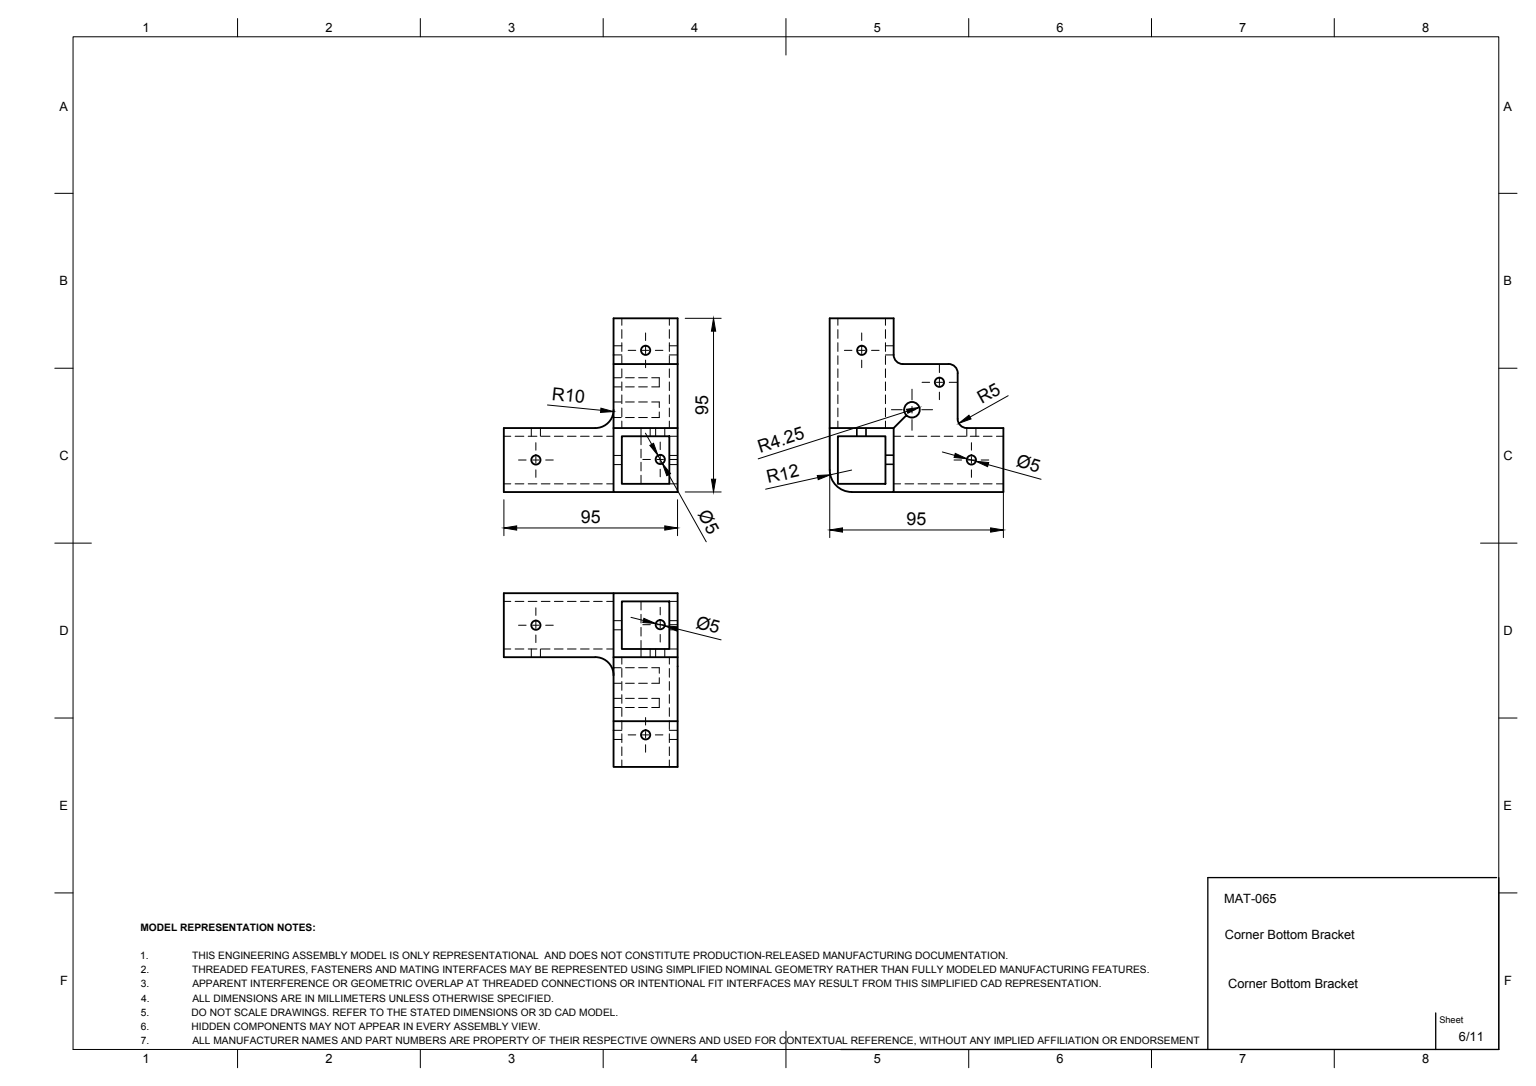
ISO-10303-21;
HEADER;
/* Generated by software containing ST-Developer
 * from STEP Tools, Inc. (www.steptools.com) 
 */

FILE_DESCRIPTION(
/* description */ (
'CAx-IF Rec.Pracs.---Representation and Presentation of Product Manufa
cturing Information (PMI)---4.0---2014-10-13'),
/* implementation_level */ '2;1');

FILE_NAME(
/* name */ 'Corner Bottom Bracket.step',
/* time_stamp */ '2026-11-15T23:28:27-08:00',
/* author */ (''),
/* organization */ (''),
/* preprocessor_version */ 'ST-DEVELOPER v20.2',
/* originating_system */ 'Autodesk Translation Framework v15.17.0.0',
/* authorisation */ '');

FILE_SCHEMA (('AUTOMOTIVE_DESIGN { 1 0 10303 214 3 1 1 }'));
ENDSEC;

DATA;
#10=MECHANICAL_DESIGN_GEOMETRIC_PRESENTATION_REPRESENTATION('',(#197),#7756);
#166=ELLIPSE('',#5063,0.0141421356237309,0.01);
#169=B_SPLINE_CURVE_WITH_KNOTS('',3,(#7622,#7623,#7624,#7625,#7626,#7627),
 .UNSPECIFIED.,.F.,.F.,(4,2,4),(-0.973960746358264,-0.811705326326323,-0.649449906294381),
 .UNSPECIFIED.);
#170=B_SPLINE_CURVE_WITH_KNOTS('',3,(#7661,#7662,#7663,#7664,#7665,#7666),
 .UNSPECIFIED.,.F.,.F.,(4,2,4),(0.649449906294381,0.811705326326323,0.973960746358265),
 .UNSPECIFIED.);
#179=SHAPE_REPRESENTATION_RELATIONSHIP('SRR','None',#7827,#188);
#188=ADVANCED_BREP_SHAPE_REPRESENTATION('',(#206),#7755);
#197=STYLED_ITEM('',(#7878),#206);
#206=MANIFOLD_SOLID_BREP('Body1',#4634);
#246=CYLINDRICAL_SURFACE('',#5062,0.01);
#247=CYLINDRICAL_SURFACE('',#5064,0.012);
#248=CYLINDRICAL_SURFACE('',#5065,0.0025);
#249=CYLINDRICAL_SURFACE('',#5066,0.0025);
#250=CYLINDRICAL_SURFACE('',#5067,0.0025);
#251=CYLINDRICAL_SURFACE('',#5068,0.0025);
#252=CYLINDRICAL_SURFACE('',#5069,0.0025);
#253=CYLINDRICAL_SURFACE('',#5070,0.0025);
#254=CYLINDRICAL_SURFACE('',#5071,0.0025);
#255=CYLINDRICAL_SURFACE('',#5072,0.0025);
#256=CYLINDRICAL_SURFACE('',#5075,0.0025);
#257=CYLINDRICAL_SURFACE('',#5078,0.00425);
#258=CYLINDRICAL_SURFACE('',#5081,0.01);
#259=CYLINDRICAL_SURFACE('',#5082,0.005);
#260=CYLINDRICAL_SURFACE('',#5083,0.005);
#261=CYLINDRICAL_SURFACE('',#5084,0.005);
#262=CYLINDRICAL_SURFACE('',#5092,0.0025);
#263=CYLINDRICAL_SURFACE('',#5093,0.0025);
#342=CIRCLE('',#5005,0.005);
#343=CIRCLE('',#5006,0.005);
#344=CIRCLE('',#5007,0.012);
#345=CIRCLE('',#5008,0.005);
#346=CIRCLE('',#5009,0.0025);
#347=CIRCLE('',#5010,0.0025);
#348=CIRCLE('',#5012,0.0025);
#349=CIRCLE('',#5013,0.0025);
#350=CIRCLE('',#5015,0.0025);
#351=CIRCLE('',#5016,0.0025);
#352=CIRCLE('',#5018,0.012);
#353=CIRCLE('',#5022,0.01);
#354=CIRCLE('',#5024,0.01);
#355=CIRCLE('',#5026,0.005);
#356=CIRCLE('',#5027,0.005);
#357=CIRCLE('',#5028,0.00425);
#358=CIRCLE('',#5029,0.005);
#359=CIRCLE('',#5030,0.0025);
#360=CIRCLE('',#5031,0.0025);
#361=CIRCLE('',#5032,0.0025);
#362=CIRCLE('',#5034,0.0025);
#363=CIRCLE('',#5036,0.0025);
#364=CIRCLE('',#5038,0.0025);
#365=CIRCLE('',#5041,0.0025);
#366=CIRCLE('',#5043,0.0025);
#367=CIRCLE('',#5045,0.0025);
#368=CIRCLE('',#5047,0.0025);
#369=CIRCLE('',#5049,0.0025);
#370=CIRCLE('',#5051,0.0025);
#371=CIRCLE('',#5054,0.0025);
#372=CIRCLE('',#5056,0.0025);
#373=CIRCLE('',#5060,0.0025);
#374=CIRCLE('',#5076,0.0025);
#375=CIRCLE('',#5079,0.00425);
#376=CIRCLE('',#5086,0.0025);
#377=CIRCLE('',#5088,0.0025);
#429=FACE_BOUND('',#917,.T.);
#430=FACE_BOUND('',#918,.T.);
#431=FACE_BOUND('',#919,.T.);
#432=FACE_BOUND('',#923,.T.);
#433=FACE_BOUND('',#925,.T.);
#434=FACE_BOUND('',#927,.T.);
#435=FACE_BOUND('',#931,.T.);
#436=FACE_BOUND('',#932,.T.);
#437=FACE_BOUND('',#933,.T.);
#438=FACE_BOUND('',#935,.T.);
#439=FACE_BOUND('',#937,.T.);
#440=FACE_BOUND('',#939,.T.);
#441=FACE_BOUND('',#942,.T.);
#442=FACE_BOUND('',#944,.T.);
#443=FACE_BOUND('',#946,.T.);
#444=FACE_BOUND('',#948,.T.);
#445=FACE_BOUND('',#950,.T.);
#446=FACE_BOUND('',#952,.T.);
#447=FACE_BOUND('',#955,.T.);
#448=FACE_BOUND('',#957,.T.);
#449=FACE_BOUND('',#961,.T.);
#450=FACE_BOUND('',#984,.T.);
#451=FACE_BOUND('',#986,.T.);
#632=FACE_OUTER_BOUND('',#916,.T.);
#633=FACE_OUTER_BOUND('',#920,.T.);
#634=FACE_OUTER_BOUND('',#921,.T.);
#635=FACE_OUTER_BOUND('',#922,.T.);
#636=FACE_OUTER_BOUND('',#924,.T.);
#637=FACE_OUTER_BOUND('',#926,.T.);
#638=FACE_OUTER_BOUND('',#928,.T.);
#639=FACE_OUTER_BOUND('',#929,.T.);
#640=FACE_OUTER_BOUND('',#930,.T.);
#641=FACE_OUTER_BOUND('',#934,.T.);
#642=FACE_OUTER_BOUND('',#936,.T.);
#643=FACE_OUTER_BOUND('',#938,.T.);
#644=FACE_OUTER_BOUND('',#940,.T.);
#645=FACE_OUTER_BOUND('',#941,.T.);
#646=FACE_OUTER_BOUND('',#943,.T.);
#647=FACE_OUTER_BOUND('',#945,.T.);
#648=FACE_OUTER_BOUND('',#947,.T.);
#649=FACE_OUTER_BOUND('',#949,.T.);
#650=FACE_OUTER_BOUND('',#951,.T.);
#651=FACE_OUTER_BOUND('',#953,.T.);
#652=FACE_OUTER_BOUND('',#954,.T.);
#653=FACE_OUTER_BOUND('',#956,.T.);
#654=FACE_OUTER_BOUND('',#958,.T.);
#655=FACE_OUTER_BOUND('',#959,.T.);
#656=FACE_OUTER_BOUND('',#960,.T.);
#657=FACE_OUTER_BOUND('',#962,.T.);
#658=FACE_OUTER_BOUND('',#963,.T.);
#659=FACE_OUTER_BOUND('',#964,.T.);
#660=FACE_OUTER_BOUND('',#965,.T.);
#661=FACE_OUTER_BOUND('',#966,.T.);
#662=FACE_OUTER_BOUND('',#967,.T.);
#663=FACE_OUTER_BOUND('',#968,.T.);
#664=FACE_OUTER_BOUND('',#969,.T.);
#665=FACE_OUTER_BOUND('',#970,.T.);
#666=FACE_OUTER_BOUND('',#971,.T.);
#667=FACE_OUTER_BOUND('',#972,.T.);
#668=FACE_OUTER_BOUND('',#973,.T.);
#669=FACE_OUTER_BOUND('',#974,.T.);
#670=FACE_OUTER_BOUND('',#975,.T.);
#671=FACE_OUTER_BOUND('',#976,.T.);
#672=FACE_OUTER_BOUND('',#977,.T.);
#673=FACE_OUTER_BOUND('',#978,.T.);
#674=FACE_OUTER_BOUND('',#979,.T.);
#675=FACE_OUTER_BOUND('',#980,.T.);
#676=FACE_OUTER_BOUND('',#981,.T.);
#677=FACE_OUTER_BOUND('',#982,.T.);
#678=FACE_OUTER_BOUND('',#983,.T.);
#679=FACE_OUTER_BOUND('',#985,.T.);
#680=FACE_OUTER_BOUND('',#987,.T.);
#681=FACE_OUTER_BOUND('',#988,.T.);
#682=FACE_OUTER_BOUND('',#989,.T.);
#683=FACE_OUTER_BOUND('',#990,.T.);
#684=FACE_OUTER_BOUND('',#991,.T.);
#916=EDGE_LOOP('',(#3939,#3940,#3941,#3942,#3943,#3944,#3945,#3946,#3947,
#3948,#3949,#3950));
#917=EDGE_LOOP('',(#3951));
#918=EDGE_LOOP('',(#3952));
#919=EDGE_LOOP('',(#3953,#3954,#3955,#3956));
#920=EDGE_LOOP('',(#3957,#3958,#3959,#3960,#3961,#3962,#3963));
#921=EDGE_LOOP('',(#3964,#3965,#3966,#3967,#3968,#3969,#3970));
#922=EDGE_LOOP('',(#3971,#3972,#3973,#3974,#3975));
#923=EDGE_LOOP('',(#3976,#3977,#3978,#3979));
#924=EDGE_LOOP('',(#3980,#3981,#3982,#3983));
#925=EDGE_LOOP('',(#3984,#3985,#3986,#3987));
#926=EDGE_LOOP('',(#3988,#3989,#3990,#3991));
#927=EDGE_LOOP('',(#3992,#3993,#3994,#3995));
#928=EDGE_LOOP('',(#3996,#3997,#3998,#3999,#4000,#4001,#4002));
#929=EDGE_LOOP('',(#4003,#4004,#4005,#4006,#4007,#4008,#4009));
#930=EDGE_LOOP('',(#4010,#4011,#4012,#4013,#4014,#4015,#4016,#4017,#4018,
#4019,#4020,#4021,#4022,#4023));
#931=EDGE_LOOP('',(#4024));
#932=EDGE_LOOP('',(#4025));
#933=EDGE_LOOP('',(#4026));
#934=EDGE_LOOP('',(#4027,#4028,#4029,#4030));
#935=EDGE_LOOP('',(#4031));
#936=EDGE_LOOP('',(#4032,#4033,#4034,#4035));
#937=EDGE_LOOP('',(#4036));
#938=EDGE_LOOP('',(#4037,#4038,#4039,#4040));
#939=EDGE_LOOP('',(#4041));
#940=EDGE_LOOP('',(#4042,#4043,#4044,#4045));
#941=EDGE_LOOP('',(#4046,#4047,#4048,#4049));
#942=EDGE_LOOP('',(#4050));
#943=EDGE_LOOP('',(#4051,#4052,#4053,#4054));
#944=EDGE_LOOP('',(#4055));
#945=EDGE_LOOP('',(#4056,#4057,#4058,#4059));
#946=EDGE_LOOP('',(#4060));
#947=EDGE_LOOP('',(#4061,#4062,#4063,#4064));
#948=EDGE_LOOP('',(#4065));
#949=EDGE_LOOP('',(#4066,#4067,#4068,#4069));
#950=EDGE_LOOP('',(#4070));
#951=EDGE_LOOP('',(#4071,#4072,#4073,#4074));
#952=EDGE_LOOP('',(#4075));
#953=EDGE_LOOP('',(#4076,#4077,#4078,#4079));
#954=EDGE_LOOP('',(#4080,#4081,#4082,#4083));
#955=EDGE_LOOP('',(#4084));
#956=EDGE_LOOP('',(#4085,#4086,#4087,#4088));
#957=EDGE_LOOP('',(#4089));
#958=EDGE_LOOP('',(#4090,#4091,#4092,#4093));
#959=EDGE_LOOP('',(#4094,#4095,#4096,#4097));
#960=EDGE_LOOP('',(#4098,#4099,#4100,#4101));
#961=EDGE_LOOP('',(#4102));
#962=EDGE_LOOP('',(#4103,#4104,#4105,#4106));
#963=EDGE_LOOP('',(#4107,#4108,#4109,#4110,#4111));
#964=EDGE_LOOP('',(#4112,#4113,#4114,#4115));
#965=EDGE_LOOP('',(#4116,#4117,#4118,#4119));
#966=EDGE_LOOP('',(#4120,#4121,#4122,#4123));
#967=EDGE_LOOP('',(#4124,#4125,#4126,#4127));
#968=EDGE_LOOP('',(#4128,#4129,#4130,#4131));
#969=EDGE_LOOP('',(#4132,#4133,#4134,#4135));
#970=EDGE_LOOP('',(#4136,#4137,#4138,#4139,#4140));
#971=EDGE_LOOP('',(#4141,#4142,#4143,#4144));
#972=EDGE_LOOP('',(#4145,#4146,#4147,#4148,#4149));
#973=EDGE_LOOP('',(#4150,#4151,#4152,#4153));
#974=EDGE_LOOP('',(#4154,#4155,#4156,#4157));
#975=EDGE_LOOP('',(#4158,#4159,#4160,#4161));
#976=EDGE_LOOP('',(#4162));
#977=EDGE_LOOP('',(#4163,#4164,#4165,#4166,#4167,#4168));
#978=EDGE_LOOP('',(#4169));
#979=EDGE_LOOP('',(#4170,#4171,#4172,#4173,#4174));
#980=EDGE_LOOP('',(#4175,#4176,#4177,#4178,#4179));
#981=EDGE_LOOP('',(#4180,#4181,#4182,#4183,#4184));
#982=EDGE_LOOP('',(#4185,#4186,#4187,#4188));
#983=EDGE_LOOP('',(#4189,#4190,#4191,#4192));
#984=EDGE_LOOP('',(#4193));
#985=EDGE_LOOP('',(#4194,#4195,#4196,#4197));
#986=EDGE_LOOP('',(#4198));
#987=EDGE_LOOP('',(#4199,#4200,#4201,#4202));
#988=EDGE_LOOP('',(#4203,#4204,#4205,#4206));
#989=EDGE_LOOP('',(#4207,#4208,#4209,#4210));
#990=EDGE_LOOP('',(#4211,#4212,#4213,#4214));
#991=EDGE_LOOP('',(#4215,#4216,#4217,#4218));
#1384=LINE('',#7405,#1877);
#1385=LINE('',#7409,#1878);
#1386=LINE('',#7413,#1879);
#1387=LINE('',#7415,#1880);
#1388=LINE('',#7417,#1881);
#1389=LINE('',#7421,#1882);
#1390=LINE('',#7423,#1883);
#1391=LINE('',#7425,#1884);
#1392=LINE('',#7433,#1885);
#1393=LINE('',#7435,#1886);
#1394=LINE('',#7437,#1887);
#1395=LINE('',#7438,#1888);
#1396=LINE('',#7442,#1889);
#1397=LINE('',#7444,#1890);
#1398=LINE('',#7448,#1891);
#1399=LINE('',#7449,#1892);
#1400=LINE('',#7452,#1893);
#1401=LINE('',#7457,#1894);
#1402=LINE('',#7459,#1895);
#1403=LINE('',#7460,#1896);
#1404=LINE('',#7464,#1897);
#1405=LINE('',#7468,#1898);
#1406=LINE('',#7470,#1899);
#1407=LINE('',#7471,#1900);
#1408=LINE('',#7474,#1901);
#1409=LINE('',#7476,#1902);
#1410=LINE('',#7478,#1903);
#1411=LINE('',#7479,#1904);
#1412=LINE('',#7482,#1905);
#1413=LINE('',#7483,#1906);
#1414=LINE('',#7486,#1907);
#1415=LINE('',#7488,#1908);
#1416=LINE('',#7490,#1909);
#1417=LINE('',#7491,#1910);
#1418=LINE('',#7494,#1911);
#1419=LINE('',#7495,#1912);
#1420=LINE('',#7498,#1913);
#1421=LINE('',#7500,#1914);
#1422=LINE('',#7502,#1915);
#1423=LINE('',#7503,#1916);
#1424=LINE('',#7505,#1917);
#1425=LINE('',#7507,#1918);
#1426=LINE('',#7510,#1919);
#1427=LINE('',#7512,#1920);
#1428=LINE('',#7514,#1921);
#1429=LINE('',#7517,#1922);
#1430=LINE('',#7521,#1923);
#1431=LINE('',#7525,#1924);
#1432=LINE('',#7528,#1925);
#1433=LINE('',#7531,#1926);
#1434=LINE('',#7541,#1927);
#1435=LINE('',#7542,#1928);
#1436=LINE('',#7546,#1929);
#1437=LINE('',#7551,#1930);
#1438=LINE('',#7553,#1931);
#1439=LINE('',#7554,#1932);
#1440=LINE('',#7559,#1933);
#1441=LINE('',#7560,#1934);
#1442=LINE('',#7563,#1935);
#1443=LINE('',#7564,#1936);
#1444=LINE('',#7568,#1937);
#1445=LINE('',#7576,#1938);
#1446=LINE('',#7578,#1939);
#1447=LINE('',#7579,#1940);
#1448=LINE('',#7584,#1941);
#1449=LINE('',#7585,#1942);
#1450=LINE('',#7590,#1943);
#1451=LINE('',#7591,#1944);
#1452=LINE('',#7595,#1945);
#1453=LINE('',#7601,#1946);
#1454=LINE('',#7603,#1947);
#1455=LINE('',#7604,#1948);
#1456=LINE('',#7609,#1949);
#1457=LINE('',#7610,#1950);
#1458=LINE('',#7613,#1951);
#1459=LINE('',#7614,#1952);
#1460=LINE('',#7616,#1953);
#1461=LINE('',#7631,#1954);
#1462=LINE('',#7633,#1955);
#1463=LINE('',#7635,#1956);
#1464=LINE('',#7637,#1957);
#1465=LINE('',#7639,#1958);
#1466=LINE('',#7641,#1959);
#1467=LINE('',#7643,#1960);
#1468=LINE('',#7645,#1961);
#1469=LINE('',#7647,#1962);
#1470=LINE('',#7648,#1963);
#1471=LINE('',#7650,#1964);
#1472=LINE('',#7651,#1965);
#1473=LINE('',#7655,#1966);
#1474=LINE('',#7660,#1967);
#1475=LINE('',#7674,#1968);
#1476=LINE('',#7676,#1969);
#1477=LINE('',#7677,#1970);
#1478=LINE('',#7682,#1971);
#1479=LINE('',#7683,#1972);
#1480=LINE('',#7688,#1973);
#1481=LINE('',#7689,#1974);
#1482=LINE('',#7691,#1975);
#1483=LINE('',#7694,#1976);
#1484=LINE('',#7696,#1977);
#1877=VECTOR('',#6064,1.);
#1878=VECTOR('',#6067,1.);
#1879=VECTOR('',#6070,1.);
#1880=VECTOR('',#6071,1.);
#1881=VECTOR('',#6072,1.);
#1882=VECTOR('',#6075,1.);
#1883=VECTOR('',#6076,1.);
#1884=VECTOR('',#6077,1.);
#1885=VECTOR('',#6084,1.);
#1886=VECTOR('',#6085,1.);
#1887=VECTOR('',#6086,1.);
#1888=VECTOR('',#6087,1.);
#1889=VECTOR('',#6090,1.);
#1890=VECTOR('',#6091,1.);
#1891=VECTOR('',#6096,1.);
#1892=VECTOR('',#6097,1.);
#1893=VECTOR('',#6100,1.);
#1894=VECTOR('',#6105,1.);
#1895=VECTOR('',#6106,1.);
#1896=VECTOR('',#6107,1.);
#1897=VECTOR('',#6110,1.);
#1898=VECTOR('',#6113,1.);
#1899=VECTOR('',#6114,1.);
#1900=VECTOR('',#6115,1.);
#1901=VECTOR('',#6116,1.);
#1902=VECTOR('',#6117,1.);
#1903=VECTOR('',#6118,1.);
#1904=VECTOR('',#6119,1.);
#1905=VECTOR('',#6122,1.);
#1906=VECTOR('',#6123,1.);
#1907=VECTOR('',#6124,1.);
#1908=VECTOR('',#6125,1.);
#1909=VECTOR('',#6126,1.);
#1910=VECTOR('',#6127,1.);
#1911=VECTOR('',#6130,1.);
#1912=VECTOR('',#6131,1.);
#1913=VECTOR('',#6132,1.);
#1914=VECTOR('',#6133,1.);
#1915=VECTOR('',#6134,1.);
#1916=VECTOR('',#6135,1.);
#1917=VECTOR('',#6138,1.);
#1918=VECTOR('',#6139,1.);
#1919=VECTOR('',#6142,1.);
#1920=VECTOR('',#6145,1.);
#1921=VECTOR('',#6146,1.);
#1922=VECTOR('',#6149,1.);
#1923=VECTOR('',#6152,1.);
#1924=VECTOR('',#6155,1.);
#1925=VECTOR('',#6158,1.);
#1926=VECTOR('',#6161,1.);
#1927=VECTOR('',#6172,1.);
#1928=VECTOR('',#6173,1.);
#1929=VECTOR('',#6178,1.);
#1930=VECTOR('',#6183,1.);
#1931=VECTOR('',#6184,1.);
#1932=VECTOR('',#6185,1.);
#1933=VECTOR('',#6190,1.);
#1934=VECTOR('',#6191,1.);
#1935=VECTOR('',#6194,1.);
#1936=VECTOR('',#6195,1.);
#1937=VECTOR('',#6200,1.);
#1938=VECTOR('',#6209,1.);
#1939=VECTOR('',#6210,1.);
#1940=VECTOR('',#6211,1.);
#1941=VECTOR('',#6216,1.);
#1942=VECTOR('',#6217,1.);
#1943=VECTOR('',#6222,1.);
#1944=VECTOR('',#6223,1.);
#1945=VECTOR('',#6228,1.);
#1946=VECTOR('',#6235,1.);
#1947=VECTOR('',#6236,1.);
#1948=VECTOR('',#6237,1.);
#1949=VECTOR('',#6242,1.);
#1950=VECTOR('',#6243,1.);
#1951=VECTOR('',#6246,1.);
#1952=VECTOR('',#6247,1.);
#1953=VECTOR('',#6250,1.);
#1954=VECTOR('',#6263,0.0025);
#1955=VECTOR('',#6266,0.0025);
#1956=VECTOR('',#6269,0.0025);
#1957=VECTOR('',#6272,0.0025);
#1958=VECTOR('',#6275,0.0025);
#1959=VECTOR('',#6278,0.0025);
#1960=VECTOR('',#6281,0.0025);
#1961=VECTOR('',#6284,0.0025);
#1962=VECTOR('',#6287,1.);
#1963=VECTOR('',#6288,1.);
#1964=VECTOR('',#6291,1.);
#1965=VECTOR('',#6292,1.);
#1966=VECTOR('',#6297,0.0025);
#1967=VECTOR('',#6304,0.00425);
#1968=VECTOR('',#6317,1.);
#1969=VECTOR('',#6318,1.);
#1970=VECTOR('',#6319,1.);
#1971=VECTOR('',#6324,1.);
#1972=VECTOR('',#6325,1.);
#1973=VECTOR('',#6330,1.);
#1974=VECTOR('',#6331,1.);
#1975=VECTOR('',#6334,1.);
#1976=VECTOR('',#6339,0.0025);
#1977=VECTOR('',#6342,0.0025);
#2288=VERTEX_POINT('',#7403);
#2289=VERTEX_POINT('',#7404);
#2290=VERTEX_POINT('',#7406);
#2291=VERTEX_POINT('',#7408);
#2292=VERTEX_POINT('',#7410);
#2293=VERTEX_POINT('',#7412);
#2294=VERTEX_POINT('',#7414);
#2295=VERTEX_POINT('',#7416);
#2296=VERTEX_POINT('',#7418);
#2297=VERTEX_POINT('',#7420);
#2298=VERTEX_POINT('',#7422);
#2299=VERTEX_POINT('',#7424);
#2300=VERTEX_POINT('',#7427);
#2301=VERTEX_POINT('',#7429);
#2302=VERTEX_POINT('',#7431);
#2303=VERTEX_POINT('',#7432);
#2304=VERTEX_POINT('',#7434);
#2305=VERTEX_POINT('',#7436);
#2306=VERTEX_POINT('',#7440);
#2307=VERTEX_POINT('',#7441);
#2308=VERTEX_POINT('',#7443);
#2309=VERTEX_POINT('',#7445);
#2310=VERTEX_POINT('',#7451);
#2311=VERTEX_POINT('',#7453);
#2312=VERTEX_POINT('',#7456);
#2313=VERTEX_POINT('',#7458);
#2314=VERTEX_POINT('',#7462);
#2315=VERTEX_POINT('',#7463);
#2316=VERTEX_POINT('',#7465);
#2317=VERTEX_POINT('',#7467);
#2318=VERTEX_POINT('',#7469);
#2319=VERTEX_POINT('',#7472);
#2320=VERTEX_POINT('',#7473);
#2321=VERTEX_POINT('',#7475);
#2322=VERTEX_POINT('',#7477);
#2323=VERTEX_POINT('',#7481);
#2324=VERTEX_POINT('',#7484);
#2325=VERTEX_POINT('',#7485);
#2326=VERTEX_POINT('',#7487);
#2327=VERTEX_POINT('',#7489);
#2328=VERTEX_POINT('',#7493);
#2329=VERTEX_POINT('',#7496);
#2330=VERTEX_POINT('',#7497);
#2331=VERTEX_POINT('',#7499);
#2332=VERTEX_POINT('',#7501);
#2333=VERTEX_POINT('',#7506);
#2334=VERTEX_POINT('',#7508);
#2335=VERTEX_POINT('',#7513);
#2336=VERTEX_POINT('',#7515);
#2337=VERTEX_POINT('',#7519);
#2338=VERTEX_POINT('',#7520);
#2339=VERTEX_POINT('',#7522);
#2340=VERTEX_POINT('',#7524);
#2341=VERTEX_POINT('',#7527);
#2342=VERTEX_POINT('',#7529);
#2343=VERTEX_POINT('',#7533);
#2344=VERTEX_POINT('',#7535);
#2345=VERTEX_POINT('',#7537);
#2346=VERTEX_POINT('',#7540);
#2347=VERTEX_POINT('',#7543);
#2348=VERTEX_POINT('',#7547);
#2349=VERTEX_POINT('',#7550);
#2350=VERTEX_POINT('',#7552);
#2351=VERTEX_POINT('',#7555);
#2352=VERTEX_POINT('',#7558);
#2353=VERTEX_POINT('',#7562);
#2354=VERTEX_POINT('',#7565);
#2355=VERTEX_POINT('',#7569);
#2356=VERTEX_POINT('',#7572);
#2357=VERTEX_POINT('',#7575);
#2358=VERTEX_POINT('',#7577);
#2359=VERTEX_POINT('',#7580);
#2360=VERTEX_POINT('',#7583);
#2361=VERTEX_POINT('',#7586);
#2362=VERTEX_POINT('',#7589);
#2363=VERTEX_POINT('',#7592);
#2364=VERTEX_POINT('',#7597);
#2365=VERTEX_POINT('',#7600);
#2366=VERTEX_POINT('',#7602);
#2367=VERTEX_POINT('',#7605);
#2368=VERTEX_POINT('',#7608);
#2369=VERTEX_POINT('',#7612);
#2370=VERTEX_POINT('',#7617);
#2371=VERTEX_POINT('',#7621);
#2372=VERTEX_POINT('',#7653);
#2373=VERTEX_POINT('',#7658);
#2374=VERTEX_POINT('',#7673);
#2375=VERTEX_POINT('',#7675);
#2376=VERTEX_POINT('',#7678);
#2377=VERTEX_POINT('',#7681);
#2378=VERTEX_POINT('',#7684);
#2379=VERTEX_POINT('',#7687);
#2853=EDGE_CURVE('',#2288,#2289,#1384,.T.);
#2854=EDGE_CURVE('',#2288,#2290,#342,.F.);
#2855=EDGE_CURVE('',#2290,#2291,#1385,.T.);
#2856=EDGE_CURVE('',#2291,#2292,#343,.T.);
#2857=EDGE_CURVE('',#2292,#2293,#1386,.T.);
#2858=EDGE_CURVE('',#2293,#2294,#1387,.T.);
#2859=EDGE_CURVE('',#2295,#2294,#1388,.T.);
#2860=EDGE_CURVE('',#2295,#2296,#344,.F.);
#2861=EDGE_CURVE('',#2297,#2296,#1389,.T.);
#2862=EDGE_CURVE('',#2297,#2298,#1390,.T.);
#2863=EDGE_CURVE('',#2298,#2299,#1391,.T.);
#2864=EDGE_CURVE('',#2299,#2289,#345,.T.);
#2865=EDGE_CURVE('',#2300,#2300,#346,.T.);
#2866=EDGE_CURVE('',#2301,#2301,#347,.T.);
#2867=EDGE_CURVE('',#2302,#2303,#1392,.T.);
#2868=EDGE_CURVE('',#2303,#2304,#1393,.T.);
#2869=EDGE_CURVE('',#2305,#2304,#1394,.T.);
#2870=EDGE_CURVE('',#2302,#2305,#1395,.T.);
#2871=EDGE_CURVE('',#2306,#2307,#1396,.T.);
#2872=EDGE_CURVE('',#2307,#2308,#1397,.T.);
#2873=EDGE_CURVE('',#2309,#2308,#348,.T.);
#2874=EDGE_CURVE('',#2308,#2309,#349,.T.);
#2875=EDGE_CURVE('',#2308,#2299,#1398,.T.);
#2876=EDGE_CURVE('',#2306,#2298,#1399,.T.);
#2877=EDGE_CURVE('',#2292,#2310,#1400,.F.);
#2878=EDGE_CURVE('',#2311,#2310,#350,.T.);
#2879=EDGE_CURVE('',#2310,#2311,#351,.T.);
#2880=EDGE_CURVE('',#2310,#2312,#1401,.F.);
#2881=EDGE_CURVE('',#2312,#2313,#1402,.T.);
#2882=EDGE_CURVE('',#2313,#2293,#1403,.T.);
#2883=EDGE_CURVE('',#2314,#2315,#1404,.T.);
#2884=EDGE_CURVE('',#2315,#2316,#352,.T.);
#2885=EDGE_CURVE('',#2316,#2317,#1405,.T.);
#2886=EDGE_CURVE('',#2318,#2317,#1406,.T.);
#2887=EDGE_CURVE('',#2318,#2314,#1407,.T.);
#2888=EDGE_CURVE('',#2319,#2320,#1408,.T.);
#2889=EDGE_CURVE('',#2319,#2321,#1409,.T.);
#2890=EDGE_CURVE('',#2321,#2322,#1410,.T.);
#2891=EDGE_CURVE('',#2320,#2322,#1411,.T.);
#2892=EDGE_CURVE('',#2323,#2297,#1412,.T.);
#2893=EDGE_CURVE('',#2323,#2306,#1413,.T.);
#2894=EDGE_CURVE('',#2324,#2325,#1414,.T.);
#2895=EDGE_CURVE('',#2324,#2326,#1415,.T.);
#2896=EDGE_CURVE('',#2326,#2327,#1416,.T.);
#2897=EDGE_CURVE('',#2325,#2327,#1417,.T.);
#2898=EDGE_CURVE('',#2313,#2328,#1418,.T.);
#2899=EDGE_CURVE('',#2328,#2294,#1419,.T.);
#2900=EDGE_CURVE('',#2329,#2330,#1420,.T.);
#2901=EDGE_CURVE('',#2329,#2331,#1421,.T.);
#2902=EDGE_CURVE('',#2331,#2332,#1422,.T.);
#2903=EDGE_CURVE('',#2330,#2332,#1423,.T.);
#2904=EDGE_CURVE('',#2296,#2315,#1424,.F.);
#2905=EDGE_CURVE('',#2314,#2333,#1425,.T.);
#2906=EDGE_CURVE('',#2333,#2334,#353,.T.);
#2907=EDGE_CURVE('',#2323,#2334,#1426,.T.);
#2908=EDGE_CURVE('',#2316,#2295,#1427,.T.);
#2909=EDGE_CURVE('',#2335,#2328,#1428,.T.);
#2910=EDGE_CURVE('',#2335,#2336,#354,.T.);
#2911=EDGE_CURVE('',#2317,#2336,#1429,.T.);
#2912=EDGE_CURVE('',#2337,#2338,#1430,.T.);
#2913=EDGE_CURVE('',#2337,#2339,#355,.T.);
#2914=EDGE_CURVE('',#2339,#2340,#1431,.T.);
#2915=EDGE_CURVE('',#2340,#2307,#356,.F.);
#2916=EDGE_CURVE('',#2334,#2341,#1432,.F.);
#2917=EDGE_CURVE('',#2342,#2341,#357,.T.);
#2918=EDGE_CURVE('',#2342,#2335,#1433,.T.);
#2919=EDGE_CURVE('',#2312,#2338,#358,.F.);
#2920=EDGE_CURVE('',#2343,#2343,#359,.T.);
#2921=EDGE_CURVE('',#2344,#2344,#360,.T.);
#2922=EDGE_CURVE('',#2345,#2345,#361,.T.);
#2923=EDGE_CURVE('',#2336,#2346,#1434,.F.);
#2924=EDGE_CURVE('',#2318,#2346,#1435,.T.);
#2925=EDGE_CURVE('',#2347,#2347,#362,.T.);
#2926=EDGE_CURVE('',#2346,#2333,#1436,.T.);
#2927=EDGE_CURVE('',#2348,#2348,#363,.T.);
#2928=EDGE_CURVE('',#2349,#2329,#1437,.T.);
#2929=EDGE_CURVE('',#2349,#2350,#1438,.T.);
#2930=EDGE_CURVE('',#2350,#2331,#1439,.T.);
#2931=EDGE_CURVE('',#2351,#2351,#364,.T.);
#2932=EDGE_CURVE('',#2352,#2330,#1440,.T.);
#2933=EDGE_CURVE('',#2349,#2352,#1441,.T.);
#2934=EDGE_CURVE('',#2353,#2332,#1442,.T.);
#2935=EDGE_CURVE('',#2352,#2353,#1443,.T.);
#2936=EDGE_CURVE('',#2354,#2354,#365,.T.);
#2937=EDGE_CURVE('',#2350,#2353,#1444,.T.);
#2938=EDGE_CURVE('',#2355,#2355,#366,.T.);
#2939=EDGE_CURVE('',#2356,#2356,#367,.T.);
#2940=EDGE_CURVE('',#2357,#2324,#1445,.T.);
#2941=EDGE_CURVE('',#2357,#2358,#1446,.T.);
#2942=EDGE_CURVE('',#2358,#2326,#1447,.T.);
#2943=EDGE_CURVE('',#2359,#2359,#368,.T.);
#2944=EDGE_CURVE('',#2360,#2325,#1448,.T.);
#2945=EDGE_CURVE('',#2357,#2360,#1449,.T.);
#2946=EDGE_CURVE('',#2361,#2361,#369,.T.);
#2947=EDGE_CURVE('',#2362,#2327,#1450,.T.);
#2948=EDGE_CURVE('',#2360,#2362,#1451,.T.);
#2949=EDGE_CURVE('',#2363,#2363,#370,.T.);
#2950=EDGE_CURVE('',#2358,#2362,#1452,.T.);
#2951=EDGE_CURVE('',#2364,#2364,#371,.T.);
#2952=EDGE_CURVE('',#2365,#2319,#1453,.T.);
#2953=EDGE_CURVE('',#2365,#2366,#1454,.T.);
#2954=EDGE_CURVE('',#2366,#2321,#1455,.T.);
#2955=EDGE_CURVE('',#2367,#2367,#372,.T.);
#2956=EDGE_CURVE('',#2368,#2320,#1456,.T.);
#2957=EDGE_CURVE('',#2365,#2368,#1457,.T.);
#2958=EDGE_CURVE('',#2369,#2322,#1458,.T.);
#2959=EDGE_CURVE('',#2368,#2369,#1459,.T.);
#2960=EDGE_CURVE('',#2366,#2369,#1460,.T.);
#2961=EDGE_CURVE('',#2370,#2370,#373,.T.);
#2962=EDGE_CURVE('',#2342,#2371,#169,.F.);
#2963=EDGE_CURVE('',#2371,#2346,#166,.T.);
#2964=EDGE_CURVE('',#2301,#2363,#1461,.T.);
#2965=EDGE_CURVE('',#2359,#2344,#1462,.T.);
#2966=EDGE_CURVE('',#2300,#2354,#1463,.T.);
#2967=EDGE_CURVE('',#2351,#2345,#1464,.T.);
#2968=EDGE_CURVE('',#2367,#2348,#1465,.T.);
#2969=EDGE_CURVE('',#2355,#2311,#1466,.T.);
#2970=EDGE_CURVE('',#2370,#2347,#1467,.T.);
#2971=EDGE_CURVE('',#2361,#2309,#1468,.T.);
#2972=EDGE_CURVE('',#2289,#2340,#1469,.F.);
#2973=EDGE_CURVE('',#2339,#2288,#1470,.T.);
#2974=EDGE_CURVE('',#2338,#2291,#1471,.T.);
#2975=EDGE_CURVE('',#2290,#2337,#1472,.F.);
#2976=EDGE_CURVE('',#2372,#2372,#374,.T.);
#2977=EDGE_CURVE('',#2372,#2343,#1473,.T.);
#2978=EDGE_CURVE('',#2373,#2373,#375,.T.);
#2979=EDGE_CURVE('',#2373,#2341,#1474,.T.);
#2980=EDGE_CURVE('',#2341,#2371,#170,.T.);
#2981=EDGE_CURVE('',#2374,#2302,#1475,.T.);
#2982=EDGE_CURVE('',#2374,#2375,#1476,.T.);
#2983=EDGE_CURVE('',#2375,#2303,#1477,.T.);
#2984=EDGE_CURVE('',#2376,#2376,#376,.T.);
#2985=EDGE_CURVE('',#2377,#2305,#1478,.T.);
#2986=EDGE_CURVE('',#2374,#2377,#1479,.T.);
#2987=EDGE_CURVE('',#2378,#2378,#377,.T.);
#2988=EDGE_CURVE('',#2379,#2304,#1480,.T.);
#2989=EDGE_CURVE('',#2377,#2379,#1481,.T.);
#2990=EDGE_CURVE('',#2375,#2379,#1482,.T.);
#2991=EDGE_CURVE('',#2378,#2356,#1483,.T.);
#2992=EDGE_CURVE('',#2376,#2364,#1484,.T.);
#3939=ORIENTED_EDGE('',*,*,#2853,.F.);
#3940=ORIENTED_EDGE('',*,*,#2854,.T.);
#3941=ORIENTED_EDGE('',*,*,#2855,.T.);
#3942=ORIENTED_EDGE('',*,*,#2856,.T.);
#3943=ORIENTED_EDGE('',*,*,#2857,.T.);
#3944=ORIENTED_EDGE('',*,*,#2858,.T.);
#3945=ORIENTED_EDGE('',*,*,#2859,.F.);
#3946=ORIENTED_EDGE('',*,*,#2860,.T.);
#3947=ORIENTED_EDGE('',*,*,#2861,.F.);
#3948=ORIENTED_EDGE('',*,*,#2862,.T.);
#3949=ORIENTED_EDGE('',*,*,#2863,.T.);
#3950=ORIENTED_EDGE('',*,*,#2864,.T.);
#3951=ORIENTED_EDGE('',*,*,#2865,.T.);
#3952=ORIENTED_EDGE('',*,*,#2866,.T.);
#3953=ORIENTED_EDGE('',*,*,#2867,.T.);
#3954=ORIENTED_EDGE('',*,*,#2868,.T.);
#3955=ORIENTED_EDGE('',*,*,#2869,.F.);
#3956=ORIENTED_EDGE('',*,*,#2870,.F.);
#3957=ORIENTED_EDGE('',*,*,#2871,.T.);
#3958=ORIENTED_EDGE('',*,*,#2872,.T.);
#3959=ORIENTED_EDGE('',*,*,#2873,.F.);
#3960=ORIENTED_EDGE('',*,*,#2874,.F.);
#3961=ORIENTED_EDGE('',*,*,#2875,.T.);
#3962=ORIENTED_EDGE('',*,*,#2863,.F.);
#3963=ORIENTED_EDGE('',*,*,#2876,.F.);
#3964=ORIENTED_EDGE('',*,*,#2857,.F.);
#3965=ORIENTED_EDGE('',*,*,#2877,.T.);
#3966=ORIENTED_EDGE('',*,*,#2878,.F.);
#3967=ORIENTED_EDGE('',*,*,#2879,.F.);
#3968=ORIENTED_EDGE('',*,*,#2880,.T.);
#3969=ORIENTED_EDGE('',*,*,#2881,.T.);
#3970=ORIENTED_EDGE('',*,*,#2882,.T.);
#3971=ORIENTED_EDGE('',*,*,#2883,.T.);
#3972=ORIENTED_EDGE('',*,*,#2884,.T.);
#3973=ORIENTED_EDGE('',*,*,#2885,.T.);
#3974=ORIENTED_EDGE('',*,*,#2886,.F.);
#3975=ORIENTED_EDGE('',*,*,#2887,.T.);
#3976=ORIENTED_EDGE('',*,*,#2888,.F.);
#3977=ORIENTED_EDGE('',*,*,#2889,.T.);
#3978=ORIENTED_EDGE('',*,*,#2890,.T.);
#3979=ORIENTED_EDGE('',*,*,#2891,.F.);
#3980=ORIENTED_EDGE('',*,*,#2862,.F.);
#3981=ORIENTED_EDGE('',*,*,#2892,.F.);
#3982=ORIENTED_EDGE('',*,*,#2893,.T.);
#3983=ORIENTED_EDGE('',*,*,#2876,.T.);
#3984=ORIENTED_EDGE('',*,*,#2894,.F.);
#3985=ORIENTED_EDGE('',*,*,#2895,.T.);
#3986=ORIENTED_EDGE('',*,*,#2896,.T.);
#3987=ORIENTED_EDGE('',*,*,#2897,.F.);
#3988=ORIENTED_EDGE('',*,*,#2858,.F.);
#3989=ORIENTED_EDGE('',*,*,#2882,.F.);
#3990=ORIENTED_EDGE('',*,*,#2898,.T.);
#3991=ORIENTED_EDGE('',*,*,#2899,.T.);
#3992=ORIENTED_EDGE('',*,*,#2900,.F.);
#3993=ORIENTED_EDGE('',*,*,#2901,.T.);
#3994=ORIENTED_EDGE('',*,*,#2902,.T.);
#3995=ORIENTED_EDGE('',*,*,#2903,.F.);
#3996=ORIENTED_EDGE('',*,*,#2861,.T.);
#3997=ORIENTED_EDGE('',*,*,#2904,.T.);
#3998=ORIENTED_EDGE('',*,*,#2883,.F.);
#3999=ORIENTED_EDGE('',*,*,#2905,.T.);
#4000=ORIENTED_EDGE('',*,*,#2906,.T.);
#4001=ORIENTED_EDGE('',*,*,#2907,.F.);
#4002=ORIENTED_EDGE('',*,*,#2892,.T.);
#4003=ORIENTED_EDGE('',*,*,#2885,.F.);
#4004=ORIENTED_EDGE('',*,*,#2908,.T.);
#4005=ORIENTED_EDGE('',*,*,#2859,.T.);
#4006=ORIENTED_EDGE('',*,*,#2899,.F.);
#4007=ORIENTED_EDGE('',*,*,#2909,.F.);
#4008=ORIENTED_EDGE('',*,*,#2910,.T.);
#4009=ORIENTED_EDGE('',*,*,#2911,.F.);
#4010=ORIENTED_EDGE('',*,*,#2912,.F.);
#4011=ORIENTED_EDGE('',*,*,#2913,.T.);
#4012=ORIENTED_EDGE('',*,*,#2914,.T.);
#4013=ORIENTED_EDGE('',*,*,#2915,.T.);
#4014=ORIENTED_EDGE('',*,*,#2871,.F.);
#4015=ORIENTED_EDGE('',*,*,#2893,.F.);
#4016=ORIENTED_EDGE('',*,*,#2907,.T.);
#4017=ORIENTED_EDGE('',*,*,#2916,.T.);
#4018=ORIENTED_EDGE('',*,*,#2917,.F.);
#4019=ORIENTED_EDGE('',*,*,#2918,.T.);
#4020=ORIENTED_EDGE('',*,*,#2909,.T.);
#4021=ORIENTED_EDGE('',*,*,#2898,.F.);
#4022=ORIENTED_EDGE('',*,*,#2881,.F.);
#4023=ORIENTED_EDGE('',*,*,#2919,.T.);
#4024=ORIENTED_EDGE('',*,*,#2920,.F.);
#4025=ORIENTED_EDGE('',*,*,#2921,.F.);
#4026=ORIENTED_EDGE('',*,*,#2922,.F.);
#4027=ORIENTED_EDGE('',*,*,#2911,.T.);
#4028=ORIENTED_EDGE('',*,*,#2923,.T.);
#4029=ORIENTED_EDGE('',*,*,#2924,.F.);
#4030=ORIENTED_EDGE('',*,*,#2886,.T.);
#4031=ORIENTED_EDGE('',*,*,#2925,.F.);
#4032=ORIENTED_EDGE('',*,*,#2924,.T.);
#4033=ORIENTED_EDGE('',*,*,#2926,.T.);
#4034=ORIENTED_EDGE('',*,*,#2905,.F.);
#4035=ORIENTED_EDGE('',*,*,#2887,.F.);
#4036=ORIENTED_EDGE('',*,*,#2927,.F.);
#4037=ORIENTED_EDGE('',*,*,#2901,.F.);
#4038=ORIENTED_EDGE('',*,*,#2928,.F.);
#4039=ORIENTED_EDGE('',*,*,#2929,.T.);
#4040=ORIENTED_EDGE('',*,*,#2930,.T.);
#4041=ORIENTED_EDGE('',*,*,#2931,.F.);
#4042=ORIENTED_EDGE('',*,*,#2900,.T.);
#4043=ORIENTED_EDGE('',*,*,#2932,.F.);
#4044=ORIENTED_EDGE('',*,*,#2933,.F.);
#4045=ORIENTED_EDGE('',*,*,#2928,.T.);
#4046=ORIENTED_EDGE('',*,*,#2903,.T.);
#4047=ORIENTED_EDGE('',*,*,#2934,.F.);
#4048=ORIENTED_EDGE('',*,*,#2935,.F.);
#4049=ORIENTED_EDGE('',*,*,#2932,.T.);
#4050=ORIENTED_EDGE('',*,*,#2936,.T.);
#4051=ORIENTED_EDGE('',*,*,#2902,.F.);
#4052=ORIENTED_EDGE('',*,*,#2930,.F.);
#4053=ORIENTED_EDGE('',*,*,#2937,.T.);
#4054=ORIENTED_EDGE('',*,*,#2934,.T.);
#4055=ORIENTED_EDGE('',*,*,#2938,.F.);
#4056=ORIENTED_EDGE('',*,*,#2929,.F.);
#4057=ORIENTED_EDGE('',*,*,#2933,.T.);
#4058=ORIENTED_EDGE('',*,*,#2935,.T.);
#4059=ORIENTED_EDGE('',*,*,#2937,.F.);
#4060=ORIENTED_EDGE('',*,*,#2939,.F.);
#4061=ORIENTED_EDGE('',*,*,#2895,.F.);
#4062=ORIENTED_EDGE('',*,*,#2940,.F.);
#4063=ORIENTED_EDGE('',*,*,#2941,.T.);
#4064=ORIENTED_EDGE('',*,*,#2942,.T.);
#4065=ORIENTED_EDGE('',*,*,#2943,.F.);
#4066=ORIENTED_EDGE('',*,*,#2894,.T.);
#4067=ORIENTED_EDGE('',*,*,#2944,.F.);
#4068=ORIENTED_EDGE('',*,*,#2945,.F.);
#4069=ORIENTED_EDGE('',*,*,#2940,.T.);
#4070=ORIENTED_EDGE('',*,*,#2946,.T.);
#4071=ORIENTED_EDGE('',*,*,#2897,.T.);
#4072=ORIENTED_EDGE('',*,*,#2947,.F.);
#4073=ORIENTED_EDGE('',*,*,#2948,.F.);
#4074=ORIENTED_EDGE('',*,*,#2944,.T.);
#4075=ORIENTED_EDGE('',*,*,#2949,.T.);
#4076=ORIENTED_EDGE('',*,*,#2896,.F.);
#4077=ORIENTED_EDGE('',*,*,#2942,.F.);
#4078=ORIENTED_EDGE('',*,*,#2950,.T.);
#4079=ORIENTED_EDGE('',*,*,#2947,.T.);
#4080=ORIENTED_EDGE('',*,*,#2941,.F.);
#4081=ORIENTED_EDGE('',*,*,#2945,.T.);
#4082=ORIENTED_EDGE('',*,*,#2948,.T.);
#4083=ORIENTED_EDGE('',*,*,#2950,.F.);
#4084=ORIENTED_EDGE('',*,*,#2951,.F.);
#4085=ORIENTED_EDGE('',*,*,#2889,.F.);
#4086=ORIENTED_EDGE('',*,*,#2952,.F.);
#4087=ORIENTED_EDGE('',*,*,#2953,.T.);
#4088=ORIENTED_EDGE('',*,*,#2954,.T.);
#4089=ORIENTED_EDGE('',*,*,#2955,.F.);
#4090=ORIENTED_EDGE('',*,*,#2888,.T.);
#4091=ORIENTED_EDGE('',*,*,#2956,.F.);
#4092=ORIENTED_EDGE('',*,*,#2957,.F.);
#4093=ORIENTED_EDGE('',*,*,#2952,.T.);
#4094=ORIENTED_EDGE('',*,*,#2891,.T.);
#4095=ORIENTED_EDGE('',*,*,#2958,.F.);
#4096=ORIENTED_EDGE('',*,*,#2959,.F.);
#4097=ORIENTED_EDGE('',*,*,#2956,.T.);
#4098=ORIENTED_EDGE('',*,*,#2890,.F.);
#4099=ORIENTED_EDGE('',*,*,#2954,.F.);
#4100=ORIENTED_EDGE('',*,*,#2960,.T.);
#4101=ORIENTED_EDGE('',*,*,#2958,.T.);
#4102=ORIENTED_EDGE('',*,*,#2961,.F.);
#4103=ORIENTED_EDGE('',*,*,#2953,.F.);
#4104=ORIENTED_EDGE('',*,*,#2957,.T.);
#4105=ORIENTED_EDGE('',*,*,#2959,.T.);
#4106=ORIENTED_EDGE('',*,*,#2960,.F.);
#4107=ORIENTED_EDGE('',*,*,#2918,.F.);
#4108=ORIENTED_EDGE('',*,*,#2962,.T.);
#4109=ORIENTED_EDGE('',*,*,#2963,.T.);
#4110=ORIENTED_EDGE('',*,*,#2923,.F.);
#4111=ORIENTED_EDGE('',*,*,#2910,.F.);
#4112=ORIENTED_EDGE('',*,*,#2884,.F.);
#4113=ORIENTED_EDGE('',*,*,#2904,.F.);
#4114=ORIENTED_EDGE('',*,*,#2860,.F.);
#4115=ORIENTED_EDGE('',*,*,#2908,.F.);
#4116=ORIENTED_EDGE('',*,*,#2866,.F.);
#4117=ORIENTED_EDGE('',*,*,#2964,.T.);
#4118=ORIENTED_EDGE('',*,*,#2949,.F.);
#4119=ORIENTED_EDGE('',*,*,#2964,.F.);
#4120=ORIENTED_EDGE('',*,*,#2943,.T.);
#4121=ORIENTED_EDGE('',*,*,#2965,.T.);
#4122=ORIENTED_EDGE('',*,*,#2921,.T.);
#4123=ORIENTED_EDGE('',*,*,#2965,.F.);
#4124=ORIENTED_EDGE('',*,*,#2865,.F.);
#4125=ORIENTED_EDGE('',*,*,#2966,.T.);
#4126=ORIENTED_EDGE('',*,*,#2936,.F.);
#4127=ORIENTED_EDGE('',*,*,#2966,.F.);
#4128=ORIENTED_EDGE('',*,*,#2931,.T.);
#4129=ORIENTED_EDGE('',*,*,#2967,.T.);
#4130=ORIENTED_EDGE('',*,*,#2922,.T.);
#4131=ORIENTED_EDGE('',*,*,#2967,.F.);
#4132=ORIENTED_EDGE('',*,*,#2955,.T.);
#4133=ORIENTED_EDGE('',*,*,#2968,.T.);
#4134=ORIENTED_EDGE('',*,*,#2927,.T.);
#4135=ORIENTED_EDGE('',*,*,#2968,.F.);
#4136=ORIENTED_EDGE('',*,*,#2938,.T.);
#4137=ORIENTED_EDGE('',*,*,#2969,.T.);
#4138=ORIENTED_EDGE('',*,*,#2878,.T.);
#4139=ORIENTED_EDGE('',*,*,#2879,.T.);
#4140=ORIENTED_EDGE('',*,*,#2969,.F.);
#4141=ORIENTED_EDGE('',*,*,#2961,.T.);
#4142=ORIENTED_EDGE('',*,*,#2970,.T.);
#4143=ORIENTED_EDGE('',*,*,#2925,.T.);
#4144=ORIENTED_EDGE('',*,*,#2970,.F.);
#4145=ORIENTED_EDGE('',*,*,#2946,.F.);
#4146=ORIENTED_EDGE('',*,*,#2971,.T.);
#4147=ORIENTED_EDGE('',*,*,#2873,.T.);
#4148=ORIENTED_EDGE('',*,*,#2874,.T.);
#4149=ORIENTED_EDGE('',*,*,#2971,.F.);
#4150=ORIENTED_EDGE('',*,*,#2853,.T.);
#4151=ORIENTED_EDGE('',*,*,#2972,.T.);
#4152=ORIENTED_EDGE('',*,*,#2914,.F.);
#4153=ORIENTED_EDGE('',*,*,#2973,.T.);
#4154=ORIENTED_EDGE('',*,*,#2912,.T.);
#4155=ORIENTED_EDGE('',*,*,#2974,.T.);
#4156=ORIENTED_EDGE('',*,*,#2855,.F.);
#4157=ORIENTED_EDGE('',*,*,#2975,.T.);
#4158=ORIENTED_EDGE('',*,*,#2976,.F.);
#4159=ORIENTED_EDGE('',*,*,#2977,.T.);
#4160=ORIENTED_EDGE('',*,*,#2920,.T.);
#4161=ORIENTED_EDGE('',*,*,#2977,.F.);
#4162=ORIENTED_EDGE('',*,*,#2976,.T.);
#4163=ORIENTED_EDGE('',*,*,#2978,.F.);
#4164=ORIENTED_EDGE('',*,*,#2979,.T.);
#4165=ORIENTED_EDGE('',*,*,#2980,.T.);
#4166=ORIENTED_EDGE('',*,*,#2962,.F.);
#4167=ORIENTED_EDGE('',*,*,#2917,.T.);
#4168=ORIENTED_EDGE('',*,*,#2979,.F.);
#4169=ORIENTED_EDGE('',*,*,#2978,.T.);
#4170=ORIENTED_EDGE('',*,*,#2980,.F.);
#4171=ORIENTED_EDGE('',*,*,#2916,.F.);
#4172=ORIENTED_EDGE('',*,*,#2906,.F.);
#4173=ORIENTED_EDGE('',*,*,#2926,.F.);
#4174=ORIENTED_EDGE('',*,*,#2963,.F.);
#4175=ORIENTED_EDGE('',*,*,#2915,.F.);
#4176=ORIENTED_EDGE('',*,*,#2972,.F.);
#4177=ORIENTED_EDGE('',*,*,#2864,.F.);
#4178=ORIENTED_EDGE('',*,*,#2875,.F.);
#4179=ORIENTED_EDGE('',*,*,#2872,.F.);
#4180=ORIENTED_EDGE('',*,*,#2880,.F.);
#4181=ORIENTED_EDGE('',*,*,#2877,.F.);
#4182=ORIENTED_EDGE('',*,*,#2856,.F.);
#4183=ORIENTED_EDGE('',*,*,#2974,.F.);
#4184=ORIENTED_EDGE('',*,*,#2919,.F.);
#4185=ORIENTED_EDGE('',*,*,#2913,.F.);
#4186=ORIENTED_EDGE('',*,*,#2975,.F.);
#4187=ORIENTED_EDGE('',*,*,#2854,.F.);
#4188=ORIENTED_EDGE('',*,*,#2973,.F.);
#4189=ORIENTED_EDGE('',*,*,#2867,.F.);
#4190=ORIENTED_EDGE('',*,*,#2981,.F.);
#4191=ORIENTED_EDGE('',*,*,#2982,.T.);
#4192=ORIENTED_EDGE('',*,*,#2983,.T.);
#4193=ORIENTED_EDGE('',*,*,#2984,.F.);
#4194=ORIENTED_EDGE('',*,*,#2870,.T.);
#4195=ORIENTED_EDGE('',*,*,#2985,.F.);
#4196=ORIENTED_EDGE('',*,*,#2986,.F.);
#4197=ORIENTED_EDGE('',*,*,#2981,.T.);
#4198=ORIENTED_EDGE('',*,*,#2987,.T.);
#4199=ORIENTED_EDGE('',*,*,#2869,.T.);
#4200=ORIENTED_EDGE('',*,*,#2988,.F.);
#4201=ORIENTED_EDGE('',*,*,#2989,.F.);
#4202=ORIENTED_EDGE('',*,*,#2985,.T.);
#4203=ORIENTED_EDGE('',*,*,#2868,.F.);
#4204=ORIENTED_EDGE('',*,*,#2983,.F.);
#4205=ORIENTED_EDGE('',*,*,#2990,.T.);
#4206=ORIENTED_EDGE('',*,*,#2988,.T.);
#4207=ORIENTED_EDGE('',*,*,#2982,.F.);
#4208=ORIENTED_EDGE('',*,*,#2986,.T.);
#4209=ORIENTED_EDGE('',*,*,#2989,.T.);
#4210=ORIENTED_EDGE('',*,*,#2990,.F.);
#4211=ORIENTED_EDGE('',*,*,#2987,.F.);
#4212=ORIENTED_EDGE('',*,*,#2991,.T.);
#4213=ORIENTED_EDGE('',*,*,#2939,.T.);
#4214=ORIENTED_EDGE('',*,*,#2991,.F.);
#4215=ORIENTED_EDGE('',*,*,#2984,.T.);
#4216=ORIENTED_EDGE('',*,*,#2992,.T.);
#4217=ORIENTED_EDGE('',*,*,#2951,.T.);
#4218=ORIENTED_EDGE('',*,*,#2992,.F.);
#4358=PLANE('',#5004);
#4359=PLANE('',#5011);
#4360=PLANE('',#5014);
#4361=PLANE('',#5017);
#4362=PLANE('',#5019);
#4363=PLANE('',#5020);
#4364=PLANE('',#5021);
#4365=PLANE('',#5023);
#4366=PLANE('',#5025);
#4367=PLANE('',#5033);
#4368=PLANE('',#5035);
#4369=PLANE('',#5037);
#4370=PLANE('',#5039);
#4371=PLANE('',#5040);
#4372=PLANE('',#5042);
#4373=PLANE('',#5044);
#4374=PLANE('',#5046);
#4375=PLANE('',#5048);
#4376=PLANE('',#5050);
#4377=PLANE('',#5052);
#4378=PLANE('',#5053);
#4379=PLANE('',#5055);
#4380=PLANE('',#5057);
#4381=PLANE('',#5058);
#4382=PLANE('',#5059);
#4383=PLANE('',#5061);
#4384=PLANE('',#5073);
#4385=PLANE('',#5074);
#4386=PLANE('',#5077);
#4387=PLANE('',#5080);
#4388=PLANE('',#5085);
#4389=PLANE('',#5087);
#4390=PLANE('',#5089);
#4391=PLANE('',#5090);
#4392=PLANE('',#5091);
#4573=ADVANCED_FACE('',(#632,#429,#430,#431),#4358,.F.);
#4574=ADVANCED_FACE('',(#633),#4359,.T.);
#4575=ADVANCED_FACE('',(#634),#4360,.F.);
#4576=ADVANCED_FACE('',(#635,#432),#4361,.T.);
#4577=ADVANCED_FACE('',(#636,#433),#4362,.T.);
#4578=ADVANCED_FACE('',(#637,#434),#4363,.T.);
#4579=ADVANCED_FACE('',(#638),#4364,.F.);
#4580=ADVANCED_FACE('',(#639),#4365,.F.);
#4581=ADVANCED_FACE('',(#640,#435,#436,#437),#4366,.T.);
#4582=ADVANCED_FACE('',(#641,#438),#4367,.T.);
#4583=ADVANCED_FACE('',(#642,#439),#4368,.F.);
#4584=ADVANCED_FACE('',(#643,#440),#4369,.T.);
#4585=ADVANCED_FACE('',(#644),#4370,.F.);
#4586=ADVANCED_FACE('',(#645,#441),#4371,.F.);
#4587=ADVANCED_FACE('',(#646,#442),#4372,.T.);
#4588=ADVANCED_FACE('',(#647,#443),#4373,.T.);
#4589=ADVANCED_FACE('',(#648,#444),#4374,.T.);
#4590=ADVANCED_FACE('',(#649,#445),#4375,.F.);
#4591=ADVANCED_FACE('',(#650,#446),#4376,.F.);
#4592=ADVANCED_FACE('',(#651),#4377,.T.);
#4593=ADVANCED_FACE('',(#652,#447),#4378,.T.);
#4594=ADVANCED_FACE('',(#653,#448),#4379,.T.);
#4595=ADVANCED_FACE('',(#654),#4380,.F.);
#4596=ADVANCED_FACE('',(#655),#4381,.F.);
#4597=ADVANCED_FACE('',(#656,#449),#4382,.T.);
#4598=ADVANCED_FACE('',(#657),#4383,.T.);
#4599=ADVANCED_FACE('',(#658),#246,.F.);
#4600=ADVANCED_FACE('',(#659),#247,.T.);
#4601=ADVANCED_FACE('',(#660),#248,.F.);
#4602=ADVANCED_FACE('',(#661),#249,.F.);
#4603=ADVANCED_FACE('',(#662),#250,.F.);
#4604=ADVANCED_FACE('',(#663),#251,.F.);
#4605=ADVANCED_FACE('',(#664),#252,.F.);
#4606=ADVANCED_FACE('',(#665),#253,.F.);
#4607=ADVANCED_FACE('',(#666),#254,.F.);
#4608=ADVANCED_FACE('',(#667),#255,.F.);
#4609=ADVANCED_FACE('',(#668),#4384,.T.);
#4610=ADVANCED_FACE('',(#669),#4385,.T.);
#4611=ADVANCED_FACE('',(#670),#256,.F.);
#4612=ADVANCED_FACE('',(#671),#4386,.T.);
#4613=ADVANCED_FACE('',(#672),#257,.F.);
#4614=ADVANCED_FACE('',(#673),#4387,.T.);
#4615=ADVANCED_FACE('',(#674),#258,.F.);
#4616=ADVANCED_FACE('',(#675),#259,.F.);
#4617=ADVANCED_FACE('',(#676),#260,.F.);
#4618=ADVANCED_FACE('',(#677),#261,.T.);
#4619=ADVANCED_FACE('',(#678,#450),#4388,.T.);
#4620=ADVANCED_FACE('',(#679,#451),#4389,.F.);
#4621=ADVANCED_FACE('',(#680),#4390,.F.);
#4622=ADVANCED_FACE('',(#681),#4391,.T.);
#4623=ADVANCED_FACE('',(#682),#4392,.T.);
#4624=ADVANCED_FACE('',(#683),#262,.F.);
#4625=ADVANCED_FACE('',(#684),#263,.F.);
#4634=CLOSED_SHELL('',(#4573,#4574,#4575,#4576,#4577,#4578,#4579,#4580,
#4581,#4582,#4583,#4584,#4585,#4586,#4587,#4588,#4589,#4590,#4591,#4592,
#4593,#4594,#4595,#4596,#4597,#4598,#4599,#4600,#4601,#4602,#4603,#4604,
#4605,#4606,#4607,#4608,#4609,#4610,#4611,#4612,#4613,#4614,#4615,#4616,
#4617,#4618,#4619,#4620,#4621,#4622,#4623,#4624,#4625));
#5003=AXIS2_PLACEMENT_3D('',#7401,#6060,#6061);
#5004=AXIS2_PLACEMENT_3D('',#7402,#6062,#6063);
#5005=AXIS2_PLACEMENT_3D('',#7407,#6065,#6066);
#5006=AXIS2_PLACEMENT_3D('',#7411,#6068,#6069);
#5007=AXIS2_PLACEMENT_3D('',#7419,#6073,#6074);
#5008=AXIS2_PLACEMENT_3D('',#7426,#6078,#6079);
#5009=AXIS2_PLACEMENT_3D('',#7428,#6080,#6081);
#5010=AXIS2_PLACEMENT_3D('',#7430,#6082,#6083);
#5011=AXIS2_PLACEMENT_3D('',#7439,#6088,#6089);
#5012=AXIS2_PLACEMENT_3D('',#7446,#6092,#6093);
#5013=AXIS2_PLACEMENT_3D('',#7447,#6094,#6095);
#5014=AXIS2_PLACEMENT_3D('',#7450,#6098,#6099);
#5015=AXIS2_PLACEMENT_3D('',#7454,#6101,#6102);
#5016=AXIS2_PLACEMENT_3D('',#7455,#6103,#6104);
#5017=AXIS2_PLACEMENT_3D('',#7461,#6108,#6109);
#5018=AXIS2_PLACEMENT_3D('',#7466,#6111,#6112);
#5019=AXIS2_PLACEMENT_3D('',#7480,#6120,#6121);
#5020=AXIS2_PLACEMENT_3D('',#7492,#6128,#6129);
#5021=AXIS2_PLACEMENT_3D('',#7504,#6136,#6137);
#5022=AXIS2_PLACEMENT_3D('',#7509,#6140,#6141);
#5023=AXIS2_PLACEMENT_3D('',#7511,#6143,#6144);
#5024=AXIS2_PLACEMENT_3D('',#7516,#6147,#6148);
#5025=AXIS2_PLACEMENT_3D('',#7518,#6150,#6151);
#5026=AXIS2_PLACEMENT_3D('',#7523,#6153,#6154);
#5027=AXIS2_PLACEMENT_3D('',#7526,#6156,#6157);
#5028=AXIS2_PLACEMENT_3D('',#7530,#6159,#6160);
#5029=AXIS2_PLACEMENT_3D('',#7532,#6162,#6163);
#5030=AXIS2_PLACEMENT_3D('',#7534,#6164,#6165);
#5031=AXIS2_PLACEMENT_3D('',#7536,#6166,#6167);
#5032=AXIS2_PLACEMENT_3D('',#7538,#6168,#6169);
#5033=AXIS2_PLACEMENT_3D('',#7539,#6170,#6171);
#5034=AXIS2_PLACEMENT_3D('',#7544,#6174,#6175);
#5035=AXIS2_PLACEMENT_3D('',#7545,#6176,#6177);
#5036=AXIS2_PLACEMENT_3D('',#7548,#6179,#6180);
#5037=AXIS2_PLACEMENT_3D('',#7549,#6181,#6182);
#5038=AXIS2_PLACEMENT_3D('',#7556,#6186,#6187);
#5039=AXIS2_PLACEMENT_3D('',#7557,#6188,#6189);
#5040=AXIS2_PLACEMENT_3D('',#7561,#6192,#6193);
#5041=AXIS2_PLACEMENT_3D('',#7566,#6196,#6197);
#5042=AXIS2_PLACEMENT_3D('',#7567,#6198,#6199);
#5043=AXIS2_PLACEMENT_3D('',#7570,#6201,#6202);
#5044=AXIS2_PLACEMENT_3D('',#7571,#6203,#6204);
#5045=AXIS2_PLACEMENT_3D('',#7573,#6205,#6206);
#5046=AXIS2_PLACEMENT_3D('',#7574,#6207,#6208);
#5047=AXIS2_PLACEMENT_3D('',#7581,#6212,#6213);
#5048=AXIS2_PLACEMENT_3D('',#7582,#6214,#6215);
#5049=AXIS2_PLACEMENT_3D('',#7587,#6218,#6219);
#5050=AXIS2_PLACEMENT_3D('',#7588,#6220,#6221);
#5051=AXIS2_PLACEMENT_3D('',#7593,#6224,#6225);
#5052=AXIS2_PLACEMENT_3D('',#7594,#6226,#6227);
#5053=AXIS2_PLACEMENT_3D('',#7596,#6229,#6230);
#5054=AXIS2_PLACEMENT_3D('',#7598,#6231,#6232);
#5055=AXIS2_PLACEMENT_3D('',#7599,#6233,#6234);
#5056=AXIS2_PLACEMENT_3D('',#7606,#6238,#6239);
#5057=AXIS2_PLACEMENT_3D('',#7607,#6240,#6241);
#5058=AXIS2_PLACEMENT_3D('',#7611,#6244,#6245);
#5059=AXIS2_PLACEMENT_3D('',#7615,#6248,#6249);
#5060=AXIS2_PLACEMENT_3D('',#7618,#6251,#6252);
#5061=AXIS2_PLACEMENT_3D('',#7619,#6253,#6254);
#5062=AXIS2_PLACEMENT_3D('',#7620,#6255,#6256);
#5063=AXIS2_PLACEMENT_3D('',#7628,#6257,#6258);
#5064=AXIS2_PLACEMENT_3D('',#7629,#6259,#6260);
#5065=AXIS2_PLACEMENT_3D('',#7630,#6261,#6262);
#5066=AXIS2_PLACEMENT_3D('',#7632,#6264,#6265);
#5067=AXIS2_PLACEMENT_3D('',#7634,#6267,#6268);
#5068=AXIS2_PLACEMENT_3D('',#7636,#6270,#6271);
#5069=AXIS2_PLACEMENT_3D('',#7638,#6273,#6274);
#5070=AXIS2_PLACEMENT_3D('',#7640,#6276,#6277);
#5071=AXIS2_PLACEMENT_3D('',#7642,#6279,#6280);
#5072=AXIS2_PLACEMENT_3D('',#7644,#6282,#6283);
#5073=AXIS2_PLACEMENT_3D('',#7646,#6285,#6286);
#5074=AXIS2_PLACEMENT_3D('',#7649,#6289,#6290);
#5075=AXIS2_PLACEMENT_3D('',#7652,#6293,#6294);
#5076=AXIS2_PLACEMENT_3D('',#7654,#6295,#6296);
#5077=AXIS2_PLACEMENT_3D('',#7656,#6298,#6299);
#5078=AXIS2_PLACEMENT_3D('',#7657,#6300,#6301);
#5079=AXIS2_PLACEMENT_3D('',#7659,#6302,#6303);
#5080=AXIS2_PLACEMENT_3D('',#7667,#6305,#6306);
#5081=AXIS2_PLACEMENT_3D('',#7668,#6307,#6308);
#5082=AXIS2_PLACEMENT_3D('',#7669,#6309,#6310);
#5083=AXIS2_PLACEMENT_3D('',#7670,#6311,#6312);
#5084=AXIS2_PLACEMENT_3D('',#7671,#6313,#6314);
#5085=AXIS2_PLACEMENT_3D('',#7672,#6315,#6316);
#5086=AXIS2_PLACEMENT_3D('',#7679,#6320,#6321);
#5087=AXIS2_PLACEMENT_3D('',#7680,#6322,#6323);
#5088=AXIS2_PLACEMENT_3D('',#7685,#6326,#6327);
#5089=AXIS2_PLACEMENT_3D('',#7686,#6328,#6329);
#5090=AXIS2_PLACEMENT_3D('',#7690,#6332,#6333);
#5091=AXIS2_PLACEMENT_3D('',#7692,#6335,#6336);
#5092=AXIS2_PLACEMENT_3D('',#7693,#6337,#6338);
#5093=AXIS2_PLACEMENT_3D('',#7695,#6340,#6341);
#6060=DIRECTION('axis',(0.,0.,1.));
#6061=DIRECTION('refdir',(1.,0.,0.));
#6062=DIRECTION('center_axis',(0.,0.,1.));
#6063=DIRECTION('ref_axis',(1.,0.,0.));
#6064=DIRECTION('',(-1.,0.,0.));
#6065=DIRECTION('center_axis',(0.,0.,1.));
#6066=DIRECTION('ref_axis',(1.,0.,0.));
#6067=DIRECTION('',(0.,-1.,0.));
#6068=DIRECTION('center_axis',(0.,0.,1.));
#6069=DIRECTION('ref_axis',(1.,0.,0.));
#6070=DIRECTION('',(1.,0.,0.));
#6071=DIRECTION('',(0.,-1.,0.));
#6072=DIRECTION('',(1.,0.,0.));
#6073=DIRECTION('center_axis',(0.,0.,1.));
#6074=DIRECTION('ref_axis',(1.,0.,0.));
#6075=DIRECTION('',(6.12323399573677E-17,-1.,0.));
#6076=DIRECTION('',(1.,0.,0.));
#6077=DIRECTION('',(0.,-1.,0.));
#6078=DIRECTION('center_axis',(0.,0.,1.));
#6079=DIRECTION('ref_axis',(1.,0.,0.));
#6080=DIRECTION('center_axis',(0.,0.,1.));
#6081=DIRECTION('ref_axis',(1.,0.,0.));
#6082=DIRECTION('center_axis',(0.,0.,1.));
#6083=DIRECTION('ref_axis',(1.,0.,0.));
#6084=DIRECTION('',(-1.,0.,0.));
#6085=DIRECTION('',(-2.00160401074247E-16,-1.,0.));
#6086=DIRECTION('',(-1.,0.,0.));
#6087=DIRECTION('',(-2.66880534765662E-16,-1.,0.));
#6088=DIRECTION('center_axis',(1.,0.,0.));
#6089=DIRECTION('ref_axis',(0.,0.,-1.));
#6090=DIRECTION('',(0.,-1.,0.));
#6091=DIRECTION('',(0.,4.95635278850516E-17,-1.));
#6092=DIRECTION('center_axis',(1.,0.,0.));
#6093=DIRECTION('ref_axis',(0.,0.,-1.));
#6094=DIRECTION('center_axis',(1.,0.,0.));
#6095=DIRECTION('ref_axis',(0.,0.,-1.));
#6096=DIRECTION('',(0.,4.95635278850516E-17,-1.));
#6097=DIRECTION('',(0.,0.,-1.));
#6098=DIRECTION('center_axis',(0.,-1.,0.));
#6099=DIRECTION('ref_axis',(0.,0.,-1.));
#6100=DIRECTION('',(0.,0.,-1.));
#6101=DIRECTION('center_axis',(0.,1.,0.));
#6102=DIRECTION('ref_axis',(0.,0.,1.));
#6103=DIRECTION('center_axis',(0.,1.,0.));
#6104=DIRECTION('ref_axis',(0.,0.,1.));
#6105=DIRECTION('',(0.,0.,-1.));
#6106=DIRECTION('',(1.,0.,0.));
#6107=DIRECTION('',(0.,0.,-1.));
#6108=DIRECTION('center_axis',(0.,0.,1.));
#6109=DIRECTION('ref_axis',(1.,0.,0.));
#6110=DIRECTION('',(6.12323399573677E-17,-1.,0.));
#6111=DIRECTION('center_axis',(0.,0.,1.));
#6112=DIRECTION('ref_axis',(1.,0.,0.));
#6113=DIRECTION('',(1.,0.,0.));
#6114=DIRECTION('',(0.,-1.,0.));
#6115=DIRECTION('',(-1.,0.,0.));
#6116=DIRECTION('',(2.00160401074247E-16,-1.,0.));
#6117=DIRECTION('',(1.,0.,0.));
#6118=DIRECTION('',(2.66880534765662E-16,-1.,0.));
#6119=DIRECTION('',(1.,0.,0.));
#6120=DIRECTION('center_axis',(0.,1.,0.));
#6121=DIRECTION('ref_axis',(0.,0.,1.));
#6122=DIRECTION('',(0.,0.,-1.));
#6123=DIRECTION('',(1.,0.,0.));
#6124=DIRECTION('',(0.,0.,-1.));
#6125=DIRECTION('',(-1.,0.,2.66880534765662E-16));
#6126=DIRECTION('',(0.,0.,-1.));
#6127=DIRECTION('',(-1.,0.,2.00160401074247E-16));
#6128=DIRECTION('center_axis',(1.,0.,0.));
#6129=DIRECTION('ref_axis',(0.,0.,-1.));
#6130=DIRECTION('',(0.,-1.,0.));
#6131=DIRECTION('',(0.,0.,-1.));
#6132=DIRECTION('',(0.,0.,-1.));
#6133=DIRECTION('',(0.,1.,2.66880534765662E-16));
#6134=DIRECTION('',(0.,0.,-1.));
#6135=DIRECTION('',(0.,1.,2.00160401074247E-16));
#6136=DIRECTION('center_axis',(1.,6.12323399573677E-17,0.));
#6137=DIRECTION('ref_axis',(-6.12323399573677E-17,1.,0.));
#6138=DIRECTION('',(0.,0.,-1.));
#6139=DIRECTION('',(0.,0.,-1.));
#6140=DIRECTION('center_axis',(1.,6.12323399573677E-17,0.));
#6141=DIRECTION('ref_axis',(-6.12323399573677E-17,1.,0.));
#6142=DIRECTION('',(6.12323399573677E-17,-1.,0.));
#6143=DIRECTION('center_axis',(0.,1.,0.));
#6144=DIRECTION('ref_axis',(0.,0.,1.));
#6145=DIRECTION('',(0.,0.,-1.));
#6146=DIRECTION('',(1.,0.,0.));
#6147=DIRECTION('center_axis',(0.,1.,0.));
#6148=DIRECTION('ref_axis',(0.,0.,1.));
#6149=DIRECTION('',(0.,0.,-1.));
#6150=DIRECTION('center_axis',(0.,0.,1.));
#6151=DIRECTION('ref_axis',(1.,0.,0.));
#6152=DIRECTION('',(0.,-1.,0.));
#6153=DIRECTION('center_axis',(0.,0.,1.));
#6154=DIRECTION('ref_axis',(1.,0.,0.));
#6155=DIRECTION('',(-1.,0.,0.));
#6156=DIRECTION('center_axis',(0.,0.,1.));
#6157=DIRECTION('ref_axis',(1.,0.,0.));
#6158=DIRECTION('',(-1.,0.,0.));
#6159=DIRECTION('center_axis',(0.,0.,1.));
#6160=DIRECTION('ref_axis',(1.,0.,0.));
#6161=DIRECTION('',(0.,-1.,0.));
#6162=DIRECTION('center_axis',(0.,0.,1.));
#6163=DIRECTION('ref_axis',(1.,0.,0.));
#6164=DIRECTION('center_axis',(0.,0.,1.));
#6165=DIRECTION('ref_axis',(1.,0.,0.));
#6166=DIRECTION('center_axis',(0.,0.,1.));
#6167=DIRECTION('ref_axis',(1.,0.,0.));
#6168=DIRECTION('center_axis',(0.,0.,1.));
#6169=DIRECTION('ref_axis',(1.,0.,0.));
#6170=DIRECTION('center_axis',(1.,0.,0.));
#6171=DIRECTION('ref_axis',(0.,0.,-1.));
#6172=DIRECTION('',(0.,-1.,0.));
#6173=DIRECTION('',(0.,0.,-1.));
#6174=DIRECTION('center_axis',(1.,0.,0.));
#6175=DIRECTION('ref_axis',(0.,0.,-1.));
#6176=DIRECTION('center_axis',(0.,-1.,0.));
#6177=DIRECTION('ref_axis',(0.,0.,-1.));
#6178=DIRECTION('',(-1.,0.,0.));
#6179=DIRECTION('center_axis',(0.,1.,0.));
#6180=DIRECTION('ref_axis',(0.,0.,1.));
#6181=DIRECTION('center_axis',(0.,2.66880534765662E-16,-1.));
#6182=DIRECTION('ref_axis',(0.,1.,2.66880534765662E-16));
#6183=DIRECTION('',(1.,0.,0.));
#6184=DIRECTION('',(0.,1.,2.66880534765662E-16));
#6185=DIRECTION('',(1.,0.,0.));
#6186=DIRECTION('center_axis',(0.,2.66880534765662E-16,-1.));
#6187=DIRECTION('ref_axis',(0.,1.,2.66880534765662E-16));
#6188=DIRECTION('center_axis',(0.,-1.,0.));
#6189=DIRECTION('ref_axis',(0.,0.,-1.));
#6190=DIRECTION('',(1.,0.,0.));
#6191=DIRECTION('',(0.,0.,-1.));
#6192=DIRECTION('center_axis',(0.,2.00160401074247E-16,-1.));
#6193=DIRECTION('ref_axis',(0.,1.,2.00160401074247E-16));
#6194=DIRECTION('',(1.,0.,0.));
#6195=DIRECTION('',(0.,1.,2.00160401074247E-16));
#6196=DIRECTION('center_axis',(0.,2.00160401074247E-16,-1.));
#6197=DIRECTION('ref_axis',(0.,1.,2.00160401074247E-16));
#6198=DIRECTION('center_axis',(0.,-1.,0.));
#6199=DIRECTION('ref_axis',(0.,0.,-1.));
#6200=DIRECTION('',(0.,0.,-1.));
#6201=DIRECTION('center_axis',(0.,-1.,0.));
#6202=DIRECTION('ref_axis',(0.,0.,-1.));
#6203=DIRECTION('center_axis',(1.,0.,0.));
#6204=DIRECTION('ref_axis',(0.,1.,0.));
#6205=DIRECTION('center_axis',(1.,0.,0.));
#6206=DIRECTION('ref_axis',(0.,0.,-1.));
#6207=DIRECTION('center_axis',(-2.66880534765662E-16,0.,-1.));
#6208=DIRECTION('ref_axis',(-1.,0.,2.66880534765662E-16));
#6209=DIRECTION('',(0.,1.,0.));
#6210=DIRECTION('',(-1.,0.,2.66880534765662E-16));
#6211=DIRECTION('',(0.,1.,0.));
#6212=DIRECTION('center_axis',(-2.66880534765662E-16,0.,-1.));
#6213=DIRECTION('ref_axis',(-1.,0.,2.66880534765662E-16));
#6214=DIRECTION('center_axis',(1.,0.,0.));
#6215=DIRECTION('ref_axis',(0.,0.,-1.));
#6216=DIRECTION('',(0.,1.,0.));
#6217=DIRECTION('',(0.,0.,-1.));
#6218=DIRECTION('center_axis',(1.,0.,0.));
#6219=DIRECTION('ref_axis',(0.,0.,-1.));
#6220=DIRECTION('center_axis',(-2.00160401074247E-16,0.,-1.));
#6221=DIRECTION('ref_axis',(-1.,0.,2.00160401074247E-16));
#6222=DIRECTION('',(0.,1.,0.));
#6223=DIRECTION('',(-1.,0.,2.00160401074247E-16));
#6224=DIRECTION('center_axis',(-2.00160401074247E-16,0.,-1.));
#6225=DIRECTION('ref_axis',(-1.,0.,2.00160401074247E-16));
#6226=DIRECTION('center_axis',(1.,0.,0.));
#6227=DIRECTION('ref_axis',(0.,0.,-1.));
#6228=DIRECTION('',(0.,0.,-1.));
#6229=DIRECTION('center_axis',(0.,1.,0.));
#6230=DIRECTION('ref_axis',(-1.,0.,0.));
#6231=DIRECTION('center_axis',(0.,1.,0.));
#6232=DIRECTION('ref_axis',(0.,0.,1.));
#6233=DIRECTION('center_axis',(0.,-1.,0.));
#6234=DIRECTION('ref_axis',(0.,0.,-1.));
#6235=DIRECTION('',(0.,0.,1.));
#6236=DIRECTION('',(1.,0.,0.));
#6237=DIRECTION('',(0.,0.,1.));
#6238=DIRECTION('center_axis',(0.,-1.,0.));
#6239=DIRECTION('ref_axis',(0.,0.,-1.));
#6240=DIRECTION('center_axis',(-1.,-2.00160401074247E-16,0.));
#6241=DIRECTION('ref_axis',(2.00160401074247E-16,-1.,0.));
#6242=DIRECTION('',(0.,0.,1.));
#6243=DIRECTION('',(2.00160401074247E-16,-1.,0.));
#6244=DIRECTION('center_axis',(0.,-1.,0.));
#6245=DIRECTION('ref_axis',(0.,0.,-1.));
#6246=DIRECTION('',(0.,0.,1.));
#6247=DIRECTION('',(1.,0.,0.));
#6248=DIRECTION('center_axis',(-1.,-2.66880534765662E-16,0.));
#6249=DIRECTION('ref_axis',(2.66880534765662E-16,-1.,0.));
#6250=DIRECTION('',(2.66880534765662E-16,-1.,0.));
#6251=DIRECTION('center_axis',(-1.,-2.66880534765662E-16,0.));
#6252=DIRECTION('ref_axis',(2.66880534765662E-16,-1.,0.));
#6253=DIRECTION('center_axis',(0.,0.,1.));
#6254=DIRECTION('ref_axis',(1.,0.,0.));
#6255=DIRECTION('center_axis',(0.,1.,0.));
#6256=DIRECTION('ref_axis',(0.,0.,1.));
#6257=DIRECTION('center_axis',(-0.707106781186548,0.707106781186548,0.));
#6258=DIRECTION('ref_axis',(0.707106781186547,0.707106781186547,0.));
#6259=DIRECTION('center_axis',(0.,0.,-1.));
#6260=DIRECTION('ref_axis',(-1.,0.,0.));
#6261=DIRECTION('center_axis',(0.,0.,1.));
#6262=DIRECTION('ref_axis',(1.,0.,0.));
#6263=DIRECTION('',(0.,0.,1.));
#6264=DIRECTION('center_axis',(0.,0.,1.));
#6265=DIRECTION('ref_axis',(1.,0.,0.));
#6266=DIRECTION('',(0.,0.,1.));
#6267=DIRECTION('center_axis',(0.,0.,1.));
#6268=DIRECTION('ref_axis',(1.,0.,0.));
#6269=DIRECTION('',(0.,0.,1.));
#6270=DIRECTION('center_axis',(0.,0.,1.));
#6271=DIRECTION('ref_axis',(1.,0.,0.));
#6272=DIRECTION('',(0.,0.,1.));
#6273=DIRECTION('center_axis',(0.,1.,0.));
#6274=DIRECTION('ref_axis',(0.,0.,1.));
#6275=DIRECTION('',(0.,1.,0.));
#6276=DIRECTION('center_axis',(0.,1.,0.));
#6277=DIRECTION('ref_axis',(0.,0.,1.));
#6278=DIRECTION('',(0.,1.,0.));
#6279=DIRECTION('center_axis',(1.,0.,0.));
#6280=DIRECTION('ref_axis',(0.,0.,-1.));
#6281=DIRECTION('',(1.,0.,0.));
#6282=DIRECTION('center_axis',(1.,0.,0.));
#6283=DIRECTION('ref_axis',(0.,0.,-1.));
#6284=DIRECTION('',(1.,0.,0.));
#6285=DIRECTION('center_axis',(0.,1.,4.95635278850516E-17));
#6286=DIRECTION('ref_axis',(0.,-4.95635278850516E-17,1.));
#6287=DIRECTION('',(0.,4.95635278850516E-17,-1.));
#6288=DIRECTION('',(0.,4.95635278850516E-17,-1.));
#6289=DIRECTION('center_axis',(1.,0.,0.));
#6290=DIRECTION('ref_axis',(0.,1.,0.));
#6291=DIRECTION('',(0.,0.,-1.));
#6292=DIRECTION('',(0.,4.95635278850516E-17,-1.));
#6293=DIRECTION('center_axis',(0.,0.,1.));
#6294=DIRECTION('ref_axis',(1.,0.,0.));
#6295=DIRECTION('center_axis',(0.,0.,1.));
#6296=DIRECTION('ref_axis',(1.,0.,0.));
#6297=DIRECTION('',(0.,0.,1.));
#6298=DIRECTION('center_axis',(0.,0.,1.));
#6299=DIRECTION('ref_axis',(1.,0.,0.));
#6300=DIRECTION('center_axis',(0.,0.,1.));
#6301=DIRECTION('ref_axis',(1.,0.,0.));
#6302=DIRECTION('center_axis',(0.,0.,1.));
#6303=DIRECTION('ref_axis',(1.,0.,0.));
#6304=DIRECTION('',(0.,0.,1.));
#6305=DIRECTION('center_axis',(0.,0.,1.));
#6306=DIRECTION('ref_axis',(1.,0.,0.));
#6307=DIRECTION('center_axis',(-1.,0.,0.));
#6308=DIRECTION('ref_axis',(0.,0.,1.));
#6309=DIRECTION('center_axis',(0.,-4.95635278850516E-17,1.));
#6310=DIRECTION('ref_axis',(0.,-1.,-4.95635278850516E-17));
#6311=DIRECTION('center_axis',(0.,0.,-1.));
#6312=DIRECTION('ref_axis',(-1.,0.,0.));
#6313=DIRECTION('center_axis',(0.,4.95635278850516E-17,-1.));
#6314=DIRECTION('ref_axis',(0.,1.,4.95635278850516E-17));
#6315=DIRECTION('center_axis',(0.,-1.,0.));
#6316=DIRECTION('ref_axis',(0.,0.,-1.));
#6317=DIRECTION('',(0.,0.,-1.));
#6318=DIRECTION('',(-1.,0.,0.));
#6319=DIRECTION('',(0.,0.,-1.));
#6320=DIRECTION('center_axis',(0.,-1.,0.));
#6321=DIRECTION('ref_axis',(0.,0.,-1.));
#6322=DIRECTION('center_axis',(1.,-2.66880534765662E-16,0.));
#6323=DIRECTION('ref_axis',(2.66880534765662E-16,1.,0.));
#6324=DIRECTION('',(0.,0.,-1.));
#6325=DIRECTION('',(-2.66880534765662E-16,-1.,0.));
#6326=DIRECTION('center_axis',(1.,-2.66880534765662E-16,0.));
#6327=DIRECTION('ref_axis',(2.66880534765662E-16,1.,0.));
#6328=DIRECTION('center_axis',(0.,-1.,0.));
#6329=DIRECTION('ref_axis',(0.,0.,-1.));
#6330=DIRECTION('',(0.,0.,-1.));
#6331=DIRECTION('',(-1.,0.,0.));
#6332=DIRECTION('center_axis',(1.,-2.00160401074247E-16,0.));
#6333=DIRECTION('ref_axis',(2.00160401074247E-16,1.,0.));
#6334=DIRECTION('',(-2.00160401074247E-16,-1.,0.));
#6335=DIRECTION('center_axis',(0.,0.,-1.));
#6336=DIRECTION('ref_axis',(1.,0.,0.));
#6337=DIRECTION('center_axis',(1.,0.,0.));
#6338=DIRECTION('ref_axis',(0.,0.,-1.));
#6339=DIRECTION('',(1.,0.,0.));
#6340=DIRECTION('center_axis',(0.,1.,0.));
#6341=DIRECTION('ref_axis',(0.,0.,1.));
#6342=DIRECTION('',(0.,1.,0.));
#7401=CARTESIAN_POINT('',(0.,0.,0.));
#7402=CARTESIAN_POINT('Origin',(0.0475,-0.015275768481829,0.));
#7403=CARTESIAN_POINT('',(0.065,0.00722423151817101,0.));
#7404=CARTESIAN_POINT('',(0.04,0.00722423151817101,0.));
#7405=CARTESIAN_POINT('',(0.07,0.00722423151817101,0.));
#7406=CARTESIAN_POINT('',(0.07,0.00222423151817101,0.));
#7407=CARTESIAN_POINT('Origin',(0.065,0.00222423151817101,0.));
#7408=CARTESIAN_POINT('',(0.07,-0.022775768481829,0.));
#7409=CARTESIAN_POINT('',(0.07,0.002224231518171,0.));
#7410=CARTESIAN_POINT('',(0.075,-0.027775768481829,0.));
#7411=CARTESIAN_POINT('Origin',(0.075,-0.022775768481829,0.));
#7412=CARTESIAN_POINT('',(0.095,-0.027775768481829,0.));
#7413=CARTESIAN_POINT('',(0.065,-0.027775768481829,0.));
#7414=CARTESIAN_POINT('',(0.095,-0.062775768481829,0.));
#7415=CARTESIAN_POINT('',(0.095,-0.045275768481829,0.));
#7416=CARTESIAN_POINT('',(0.012,-0.062775768481829,0.));
#7417=CARTESIAN_POINT('',(0.0475,-0.062775768481829,0.));
#7418=CARTESIAN_POINT('',(3.2225790163032E-18,-0.050775768481829,0.));
#7419=CARTESIAN_POINT('Origin',(0.012,-0.050775768481829,0.));
#7420=CARTESIAN_POINT('',(-3.46944695195361E-18,0.032224231518171,0.));
#7421=CARTESIAN_POINT('',(1.04883094781665E-18,-0.015275768481829,0.));
#7422=CARTESIAN_POINT('',(0.035,0.032224231518171,0.));
#7423=CARTESIAN_POINT('',(0.0175,0.032224231518171,0.));
#7424=CARTESIAN_POINT('',(0.035,0.012224231518171,0.));
#7425=CARTESIAN_POINT('',(0.035,0.002224231518171,0.));
#7426=CARTESIAN_POINT('Origin',(0.04,0.012224231518171,0.));
#7427=CARTESIAN_POINT('',(0.075,-0.045275768481829,0.));
#7428=CARTESIAN_POINT('Origin',(0.0775,-0.045275768481829,0.));
#7429=CARTESIAN_POINT('',(0.015,0.014724231518171,0.));
#7430=CARTESIAN_POINT('Origin',(0.0175,0.014724231518171,0.));
#7431=CARTESIAN_POINT('',(0.0305,-0.032275768481829,0.));
#7432=CARTESIAN_POINT('',(0.0045,-0.032275768481829,0.));
#7433=CARTESIAN_POINT('',(0.0175,-0.032275768481829,0.));
#7434=CARTESIAN_POINT('',(0.0045,-0.058275768481829,0.));
#7435=CARTESIAN_POINT('',(0.0045,-0.045275768481829,0.));
#7436=CARTESIAN_POINT('',(0.0305,-0.058275768481829,0.));
#7437=CARTESIAN_POINT('',(0.0175,-0.058275768481829,0.));
#7438=CARTESIAN_POINT('',(0.0305,-0.045275768481829,0.));
#7439=CARTESIAN_POINT('Origin',(0.035,0.002224231518171,0.035));
#7440=CARTESIAN_POINT('',(0.035,0.032224231518171,0.035));
#7441=CARTESIAN_POINT('',(0.035,0.012224231518171,0.035));
#7442=CARTESIAN_POINT('',(0.035,0.002224231518171,0.035));
#7443=CARTESIAN_POINT('',(0.035,0.012224231518171,0.0175));
#7444=CARTESIAN_POINT('',(0.035,0.012224231518171,0.));
#7445=CARTESIAN_POINT('',(0.035,0.014724231518171,0.02));
#7446=CARTESIAN_POINT('Origin',(0.035,0.014724231518171,0.0175));
#7447=CARTESIAN_POINT('Origin',(0.035,0.014724231518171,0.0175));
#7448=CARTESIAN_POINT('',(0.035,0.012224231518171,0.));
#7449=CARTESIAN_POINT('',(0.035,0.032224231518171,0.035));
#7450=CARTESIAN_POINT('Origin',(0.0175,-0.027775768481829,0.095));
#7451=CARTESIAN_POINT('',(0.075,-0.027775768481829,0.0175));
#7452=CARTESIAN_POINT('',(0.075,-0.027775768481829,0.095));
#7453=CARTESIAN_POINT('',(0.0775,-0.027775768481829,0.015));
#7454=CARTESIAN_POINT('Origin',(0.0775,-0.027775768481829,0.0175));
#7455=CARTESIAN_POINT('Origin',(0.0775,-0.027775768481829,0.0175));
#7456=CARTESIAN_POINT('',(0.075,-0.027775768481829,0.035));
#7457=CARTESIAN_POINT('',(0.075,-0.027775768481829,0.095));
#7458=CARTESIAN_POINT('',(0.095,-0.027775768481829,0.035));
#7459=CARTESIAN_POINT('',(0.065,-0.027775768481829,0.035));
#7460=CARTESIAN_POINT('',(0.095,-0.027775768481829,0.035));
#7461=CARTESIAN_POINT('Origin',(0.0475,-0.015275768481829,0.095));
#7462=CARTESIAN_POINT('',(1.81423519728374E-18,-0.027775768481829,0.095));
#7463=CARTESIAN_POINT('',(3.2225790163032E-18,-0.050775768481829,0.095));
#7464=CARTESIAN_POINT('',(1.04883094781665E-18,-0.015275768481829,0.095));
#7465=CARTESIAN_POINT('',(0.012,-0.062775768481829,0.095));
#7466=CARTESIAN_POINT('Origin',(0.012,-0.050775768481829,0.095));
#7467=CARTESIAN_POINT('',(0.035,-0.062775768481829,0.095));
#7468=CARTESIAN_POINT('',(0.0475,-0.062775768481829,0.095));
#7469=CARTESIAN_POINT('',(0.035,-0.027775768481829,0.095));
#7470=CARTESIAN_POINT('',(0.035,-0.045275768481829,0.095));
#7471=CARTESIAN_POINT('',(0.0175,-0.027775768481829,0.095));
#7472=CARTESIAN_POINT('',(0.0045,-0.032275768481829,0.095));
#7473=CARTESIAN_POINT('',(0.0045,-0.058275768481829,0.095));
#7474=CARTESIAN_POINT('',(0.0045,-0.045275768481829,0.095));
#7475=CARTESIAN_POINT('',(0.0305,-0.032275768481829,0.095));
#7476=CARTESIAN_POINT('',(0.0175,-0.032275768481829,0.095));
#7477=CARTESIAN_POINT('',(0.0305,-0.058275768481829,0.095));
#7478=CARTESIAN_POINT('',(0.0305,-0.045275768481829,0.095));
#7479=CARTESIAN_POINT('',(0.0175,-0.058275768481829,0.095));
#7480=CARTESIAN_POINT('Origin',(0.0175,0.032224231518171,0.035));
#7481=CARTESIAN_POINT('',(-3.46944695195361E-18,0.032224231518171,0.035));
#7482=CARTESIAN_POINT('',(-3.46944695195361E-18,0.032224231518171,0.035));
#7483=CARTESIAN_POINT('',(0.0175,0.032224231518171,0.035));
#7484=CARTESIAN_POINT('',(0.0305,0.032224231518171,0.0305));
#7485=CARTESIAN_POINT('',(0.0305,0.032224231518171,0.0045));
#7486=CARTESIAN_POINT('',(0.0305,0.032224231518171,0.0175));
#7487=CARTESIAN_POINT('',(0.0045,0.032224231518171,0.0305));
#7488=CARTESIAN_POINT('',(0.0175,0.032224231518171,0.0305));
#7489=CARTESIAN_POINT('',(0.0045,0.032224231518171,0.0045));
#7490=CARTESIAN_POINT('',(0.0045,0.032224231518171,0.0175));
#7491=CARTESIAN_POINT('',(0.0175,0.032224231518171,0.0045));
#7492=CARTESIAN_POINT('Origin',(0.095,-0.045275768481829,0.035));
#7493=CARTESIAN_POINT('',(0.095,-0.062775768481829,0.035));
#7494=CARTESIAN_POINT('',(0.095,-0.045275768481829,0.035));
#7495=CARTESIAN_POINT('',(0.095,-0.062775768481829,0.035));
#7496=CARTESIAN_POINT('',(0.095,-0.058275768481829,0.0305));
#7497=CARTESIAN_POINT('',(0.095,-0.058275768481829,0.0045));
#7498=CARTESIAN_POINT('',(0.095,-0.058275768481829,0.0175));
#7499=CARTESIAN_POINT('',(0.095,-0.032275768481829,0.0305));
#7500=CARTESIAN_POINT('',(0.095,-0.045275768481829,0.0305));
#7501=CARTESIAN_POINT('',(0.095,-0.032275768481829,0.0045));
#7502=CARTESIAN_POINT('',(0.095,-0.032275768481829,0.0175));
#7503=CARTESIAN_POINT('',(0.095,-0.045275768481829,0.0045));
#7504=CARTESIAN_POINT('Origin',(1.04883094781665E-18,-0.015275768481829,
0.035));
#7505=CARTESIAN_POINT('',(3.2225790163032E-18,-0.050775768481829,0.035));
#7506=CARTESIAN_POINT('',(1.81423519728374E-18,-0.027775768481829,0.045));
#7507=CARTESIAN_POINT('',(1.81423519728374E-18,-0.027775768481829,0.095));
#7508=CARTESIAN_POINT('',(1.20191179771007E-18,-0.017775768481829,0.035));
#7509=CARTESIAN_POINT('Origin',(0.,-0.017775768481829,0.045));
#7510=CARTESIAN_POINT('',(1.04883094781665E-18,-0.015275768481829,0.035));
#7511=CARTESIAN_POINT('Origin',(0.0475,-0.062775768481829,0.035));
#7512=CARTESIAN_POINT('',(0.012,-0.062775768481829,0.035));
#7513=CARTESIAN_POINT('',(0.045,-0.062775768481829,0.035));
#7514=CARTESIAN_POINT('',(0.0475,-0.062775768481829,0.035));
#7515=CARTESIAN_POINT('',(0.035,-0.062775768481829,0.045));
#7516=CARTESIAN_POINT('Origin',(0.045,-0.062775768481829,0.045));
#7517=CARTESIAN_POINT('',(0.035,-0.062775768481829,0.095));
#7518=CARTESIAN_POINT('Origin',(0.0475,-0.015275768481829,0.035));
#7519=CARTESIAN_POINT('',(0.07,0.00222423151817101,0.035));
#7520=CARTESIAN_POINT('',(0.07,-0.022775768481829,0.035));
#7521=CARTESIAN_POINT('',(0.07,0.002224231518171,0.035));
#7522=CARTESIAN_POINT('',(0.065,0.00722423151817101,0.035));
#7523=CARTESIAN_POINT('Origin',(0.065,0.00222423151817101,0.035));
#7524=CARTESIAN_POINT('',(0.04,0.00722423151817101,0.035));
#7525=CARTESIAN_POINT('',(0.07,0.00722423151817101,0.035));
#7526=CARTESIAN_POINT('Origin',(0.04,0.012224231518171,0.035));
#7527=CARTESIAN_POINT('',(0.04075,-0.017775768481829,0.035));
#7528=CARTESIAN_POINT('',(0.0475,-0.017775768481829,0.035));
#7529=CARTESIAN_POINT('',(0.045,-0.022025768481829,0.035));
#7530=CARTESIAN_POINT('Origin',(0.045,-0.017775768481829,0.035));
#7531=CARTESIAN_POINT('',(0.045,-0.062775768481829,0.035));
#7532=CARTESIAN_POINT('Origin',(0.075,-0.022775768481829,0.035));
#7533=CARTESIAN_POINT('',(0.0575,-0.00277576848182899,0.035));
#7534=CARTESIAN_POINT('Origin',(0.06,-0.00277576848182899,0.035));
#7535=CARTESIAN_POINT('',(0.015,0.014724231518171,0.035));
#7536=CARTESIAN_POINT('Origin',(0.0175,0.014724231518171,0.035));
#7537=CARTESIAN_POINT('',(0.075,-0.045275768481829,0.035));
#7538=CARTESIAN_POINT('Origin',(0.0775,-0.045275768481829,0.035));
#7539=CARTESIAN_POINT('Origin',(0.035,-0.045275768481829,0.095));
#7540=CARTESIAN_POINT('',(0.035,-0.027775768481829,0.045));
#7541=CARTESIAN_POINT('',(0.035,-0.027775768481829,0.045));
#7542=CARTESIAN_POINT('',(0.035,-0.027775768481829,0.095));
#7543=CARTESIAN_POINT('',(0.035,-0.045275768481829,0.08));
#7544=CARTESIAN_POINT('Origin',(0.035,-0.045275768481829,0.0775));
#7545=CARTESIAN_POINT('Origin',(0.0175,-0.027775768481829,0.095));
#7546=CARTESIAN_POINT('',(0.0175,-0.027775768481829,0.045));
#7547=CARTESIAN_POINT('',(0.0175,-0.027775768481829,0.075));
#7548=CARTESIAN_POINT('Origin',(0.0175,-0.027775768481829,0.0775));
#7549=CARTESIAN_POINT('Origin',(0.035,-0.045275768481829,0.0305));
#7550=CARTESIAN_POINT('',(0.035,-0.058275768481829,0.0305));
#7551=CARTESIAN_POINT('',(0.035,-0.058275768481829,0.0305));
#7552=CARTESIAN_POINT('',(0.035,-0.032275768481829,0.0305));
#7553=CARTESIAN_POINT('',(0.035,-0.045275768481829,0.0305));
#7554=CARTESIAN_POINT('',(0.035,-0.032275768481829,0.0305));
#7555=CARTESIAN_POINT('',(0.075,-0.045275768481829,0.0305));
#7556=CARTESIAN_POINT('Origin',(0.0775,-0.045275768481829,0.0305));
#7557=CARTESIAN_POINT('Origin',(0.035,-0.058275768481829,0.0175));
#7558=CARTESIAN_POINT('',(0.035,-0.058275768481829,0.0045));
#7559=CARTESIAN_POINT('',(0.035,-0.058275768481829,0.0045));
#7560=CARTESIAN_POINT('',(0.035,-0.058275768481829,0.0175));
#7561=CARTESIAN_POINT('Origin',(0.035,-0.045275768481829,0.0045));
#7562=CARTESIAN_POINT('',(0.035,-0.032275768481829,0.0045));
#7563=CARTESIAN_POINT('',(0.035,-0.032275768481829,0.0045));
#7564=CARTESIAN_POINT('',(0.035,-0.045275768481829,0.0045));
#7565=CARTESIAN_POINT('',(0.075,-0.045275768481829,0.0045));
#7566=CARTESIAN_POINT('Origin',(0.0775,-0.045275768481829,0.0045));
#7567=CARTESIAN_POINT('Origin',(0.035,-0.032275768481829,0.0175));
#7568=CARTESIAN_POINT('',(0.035,-0.032275768481829,0.0175));
#7569=CARTESIAN_POINT('',(0.0775,-0.032275768481829,0.015));
#7570=CARTESIAN_POINT('Origin',(0.0775,-0.032275768481829,0.0175));
#7571=CARTESIAN_POINT('Origin',(0.035,-0.045275768481829,0.0175));
#7572=CARTESIAN_POINT('',(0.035,-0.044975768481829,0.012));
#7573=CARTESIAN_POINT('Origin',(0.035,-0.044975768481829,0.0095));
#7574=CARTESIAN_POINT('Origin',(0.0175,-0.027775768481829,0.0305));
#7575=CARTESIAN_POINT('',(0.0305,-0.027775768481829,0.0305));
#7576=CARTESIAN_POINT('',(0.0305,-0.027775768481829,0.0305));
#7577=CARTESIAN_POINT('',(0.0045,-0.027775768481829,0.0305));
#7578=CARTESIAN_POINT('',(0.0175,-0.027775768481829,0.0305));
#7579=CARTESIAN_POINT('',(0.0045,-0.027775768481829,0.0305));
#7580=CARTESIAN_POINT('',(0.015,0.014724231518171,0.0305));
#7581=CARTESIAN_POINT('Origin',(0.0175,0.014724231518171,0.0305));
#7582=CARTESIAN_POINT('Origin',(0.0305,-0.027775768481829,0.0175));
#7583=CARTESIAN_POINT('',(0.0305,-0.027775768481829,0.0045));
#7584=CARTESIAN_POINT('',(0.0305,-0.027775768481829,0.0045));
#7585=CARTESIAN_POINT('',(0.0305,-0.027775768481829,0.0175));
#7586=CARTESIAN_POINT('',(0.0305,0.014724231518171,0.02));
#7587=CARTESIAN_POINT('Origin',(0.0305,0.014724231518171,0.0175));
#7588=CARTESIAN_POINT('Origin',(0.0175,-0.027775768481829,0.0045));
#7589=CARTESIAN_POINT('',(0.0045,-0.027775768481829,0.0045));
#7590=CARTESIAN_POINT('',(0.0045,-0.027775768481829,0.0045));
#7591=CARTESIAN_POINT('',(0.0175,-0.027775768481829,0.0045));
#7592=CARTESIAN_POINT('',(0.015,0.014724231518171,0.0045));
#7593=CARTESIAN_POINT('Origin',(0.0175,0.014724231518171,0.0045));
#7594=CARTESIAN_POINT('Origin',(0.0045,-0.027775768481829,0.0175));
#7595=CARTESIAN_POINT('',(0.0045,-0.027775768481829,0.0175));
#7596=CARTESIAN_POINT('Origin',(0.0175,-0.027775768481829,0.0175));
#7597=CARTESIAN_POINT('',(0.0172,-0.027775768481829,0.007));
#7598=CARTESIAN_POINT('Origin',(0.0172,-0.027775768481829,0.0095));
#7599=CARTESIAN_POINT('Origin',(0.0175,-0.032275768481829,0.035));
#7600=CARTESIAN_POINT('',(0.0045,-0.032275768481829,0.035));
#7601=CARTESIAN_POINT('',(0.0045,-0.032275768481829,0.035));
#7602=CARTESIAN_POINT('',(0.0305,-0.032275768481829,0.035));
#7603=CARTESIAN_POINT('',(0.0175,-0.032275768481829,0.035));
#7604=CARTESIAN_POINT('',(0.0305,-0.032275768481829,0.035));
#7605=CARTESIAN_POINT('',(0.0175,-0.032275768481829,0.075));
#7606=CARTESIAN_POINT('Origin',(0.0175,-0.032275768481829,0.0775));
#7607=CARTESIAN_POINT('Origin',(0.0045,-0.045275768481829,0.035));
#7608=CARTESIAN_POINT('',(0.0045,-0.058275768481829,0.035));
#7609=CARTESIAN_POINT('',(0.0045,-0.058275768481829,0.035));
#7610=CARTESIAN_POINT('',(0.0045,-0.045275768481829,0.035));
#7611=CARTESIAN_POINT('Origin',(0.0175,-0.058275768481829,0.035));
#7612=CARTESIAN_POINT('',(0.0305,-0.058275768481829,0.035));
#7613=CARTESIAN_POINT('',(0.0305,-0.058275768481829,0.035));
#7614=CARTESIAN_POINT('',(0.0175,-0.058275768481829,0.035));
#7615=CARTESIAN_POINT('Origin',(0.0305,-0.045275768481829,0.035));
#7616=CARTESIAN_POINT('',(0.0305,-0.045275768481829,0.035));
#7617=CARTESIAN_POINT('',(0.0305,-0.045275768481829,0.08));
#7618=CARTESIAN_POINT('Origin',(0.0305,-0.045275768481829,0.0775));
#7619=CARTESIAN_POINT('Origin',(0.0175,-0.045275768481829,0.035));
#7620=CARTESIAN_POINT('Origin',(0.045,-0.015275768481829,0.045));
#7621=CARTESIAN_POINT('',(0.0419947961799572,-0.0207809723018718,0.0354622460715324));
#7622=CARTESIAN_POINT('Ctrl Pts',(0.0419947961799572,-0.0207809723018718,
0.0354622460715324));
#7623=CARTESIAN_POINT('Ctrl Pts',(0.0423680832260346,-0.0211542593479493,
0.0353446288982169));
#7624=CARTESIAN_POINT('Ctrl Pts',(0.0428414808162073,-0.0214803550845837,
0.0352213771897135));
#7625=CARTESIAN_POINT('Ctrl Pts',(0.0438867716250497,-0.0219162865891378,
0.0350480458316003));
#7626=CARTESIAN_POINT('Ctrl Pts',(0.0444591485998935,-0.022025768481829,
0.035));
#7627=CARTESIAN_POINT('Ctrl Pts',(0.045,-0.022025768481829,0.035));
#7628=CARTESIAN_POINT('Origin',(0.045,-0.017775768481829,0.045));
#7629=CARTESIAN_POINT('Origin',(0.012,-0.050775768481829,0.035));
#7630=CARTESIAN_POINT('Origin',(0.0175,0.014724231518171,-0.005));
#7631=CARTESIAN_POINT('',(0.015,0.014724231518171,-0.005));
#7632=CARTESIAN_POINT('Origin',(0.0175,0.014724231518171,-0.005));
#7633=CARTESIAN_POINT('',(0.015,0.014724231518171,-0.005));
#7634=CARTESIAN_POINT('Origin',(0.0775,-0.045275768481829,-0.005));
#7635=CARTESIAN_POINT('',(0.075,-0.045275768481829,-0.005));
#7636=CARTESIAN_POINT('Origin',(0.0775,-0.045275768481829,-0.005));
#7637=CARTESIAN_POINT('',(0.075,-0.045275768481829,-0.005));
#7638=CARTESIAN_POINT('Origin',(0.0175,-0.037775768481829,0.0775));
#7639=CARTESIAN_POINT('',(0.0175,-0.037775768481829,0.075));
#7640=CARTESIAN_POINT('Origin',(0.0775,-0.037775768481829,0.0175));
#7641=CARTESIAN_POINT('',(0.0775,-0.037775768481829,0.015));
#7642=CARTESIAN_POINT('Origin',(0.025,-0.045275768481829,0.0775));
#7643=CARTESIAN_POINT('',(0.025,-0.045275768481829,0.08));
#7644=CARTESIAN_POINT('Origin',(0.025,0.014724231518171,0.0175));
#7645=CARTESIAN_POINT('',(0.025,0.014724231518171,0.02));
#7646=CARTESIAN_POINT('Origin',(0.07,0.00722423151817101,0.0175));
#7647=CARTESIAN_POINT('',(0.04,0.00722423151817101,0.035));
#7648=CARTESIAN_POINT('',(0.065,0.00722423151817101,0.0175));
#7649=CARTESIAN_POINT('Origin',(0.07,0.002224231518171,0.0175));
#7650=CARTESIAN_POINT('',(0.07,-0.022775768481829,0.0175));
#7651=CARTESIAN_POINT('',(0.07,0.002224231518171,0.0175));
#7652=CARTESIAN_POINT('Origin',(0.06,-0.00277576848182899,0.01));
#7653=CARTESIAN_POINT('',(0.0575,-0.00277576848182899,0.01));
#7654=CARTESIAN_POINT('Origin',(0.06,-0.00277576848182899,0.01));
#7655=CARTESIAN_POINT('',(0.0575,-0.00277576848182899,0.01));
#7656=CARTESIAN_POINT('Origin',(0.0475,-0.015275768481829,0.01));
#7657=CARTESIAN_POINT('Origin',(0.045,-0.017775768481829,0.01));
#7658=CARTESIAN_POINT('',(0.04075,-0.017775768481829,0.01));
#7659=CARTESIAN_POINT('Origin',(0.045,-0.017775768481829,0.01));
#7660=CARTESIAN_POINT('',(0.04075,-0.017775768481829,0.01));
#7661=CARTESIAN_POINT('Ctrl Pts',(0.04075,-0.017775768481829,0.035));
#7662=CARTESIAN_POINT('Ctrl Pts',(0.04075,-0.0183166198819355,0.035));
#7663=CARTESIAN_POINT('Ctrl Pts',(0.0408594818926913,-0.0188889968567793,
0.0350480458316003));
#7664=CARTESIAN_POINT('Ctrl Pts',(0.0412954133972453,-0.0199342876656216,
0.0352213771897135));
#7665=CARTESIAN_POINT('Ctrl Pts',(0.0416215091338797,-0.0204076852557944,
0.0353446288982169));
#7666=CARTESIAN_POINT('Ctrl Pts',(0.0419947961799572,-0.0207809723018718,
0.0354622460715324));
#7667=CARTESIAN_POINT('Origin',(0.0475,-0.015275768481829,0.01));
#7668=CARTESIAN_POINT('Origin',(0.0175,-0.017775768481829,0.045));
#7669=CARTESIAN_POINT('Origin',(0.04,0.012224231518171,0.035));
#7670=CARTESIAN_POINT('Origin',(0.075,-0.022775768481829,0.0175));
#7671=CARTESIAN_POINT('Origin',(0.065,0.00222423151817101,0.0175));
#7672=CARTESIAN_POINT('Origin',(0.0175,-0.032275768481829,0.02));
#7673=CARTESIAN_POINT('',(0.0305,-0.032275768481829,0.02));
#7674=CARTESIAN_POINT('',(0.0305,-0.032275768481829,0.02));
#7675=CARTESIAN_POINT('',(0.0045,-0.032275768481829,0.02));
#7676=CARTESIAN_POINT('',(0.0175,-0.032275768481829,0.02));
#7677=CARTESIAN_POINT('',(0.0045,-0.032275768481829,0.02));
#7678=CARTESIAN_POINT('',(0.0172,-0.032275768481829,0.007));
#7679=CARTESIAN_POINT('Origin',(0.0172,-0.032275768481829,0.0095));
#7680=CARTESIAN_POINT('Origin',(0.0305,-0.045275768481829,0.02));
#7681=CARTESIAN_POINT('',(0.0305,-0.058275768481829,0.02));
#7682=CARTESIAN_POINT('',(0.0305,-0.058275768481829,0.02));
#7683=CARTESIAN_POINT('',(0.0305,-0.045275768481829,0.02));
#7684=CARTESIAN_POINT('',(0.0305,-0.044975768481829,0.012));
#7685=CARTESIAN_POINT('Origin',(0.0305,-0.044975768481829,0.0095));
#7686=CARTESIAN_POINT('Origin',(0.0175,-0.058275768481829,0.02));
#7687=CARTESIAN_POINT('',(0.0045,-0.058275768481829,0.02));
#7688=CARTESIAN_POINT('',(0.0045,-0.058275768481829,0.02));
#7689=CARTESIAN_POINT('',(0.0175,-0.058275768481829,0.02));
#7690=CARTESIAN_POINT('Origin',(0.0045,-0.045275768481829,0.02));
#7691=CARTESIAN_POINT('',(0.0045,-0.045275768481829,0.02));
#7692=CARTESIAN_POINT('Origin',(0.0475,-0.015275768481829,0.02));
#7693=CARTESIAN_POINT('Origin',(0.005,-0.044975768481829,0.0095));
#7694=CARTESIAN_POINT('',(0.005,-0.044975768481829,0.012));
#7695=CARTESIAN_POINT('Origin',(0.0172,-0.052775768481829,0.0095));
#7696=CARTESIAN_POINT('',(0.0172,-0.052775768481829,0.007));
#7744=UNCERTAINTY_MEASURE_WITH_UNIT(LENGTH_MEASURE(1.E-5),#7757,
'DISTANCE_ACCURACY_VALUE',
'Maximum model space distance between geometric entities at asserted c
onnectivities');
#7745=UNCERTAINTY_MEASURE_WITH_UNIT(LENGTH_MEASURE(1.E-5),#7757,
'DISTANCE_ACCURACY_VALUE',
'Maximum model space distance between geometric entities at asserted c
onnectivities');
#7755=(
GEOMETRIC_REPRESENTATION_CONTEXT(3)
GLOBAL_UNCERTAINTY_ASSIGNED_CONTEXT((#7744))
GLOBAL_UNIT_ASSIGNED_CONTEXT((#7757,#7758,#7759))
REPRESENTATION_CONTEXT('','3D')
);
#7756=(
GEOMETRIC_REPRESENTATION_CONTEXT(3)
GLOBAL_UNCERTAINTY_ASSIGNED_CONTEXT((#7745))
GLOBAL_UNIT_ASSIGNED_CONTEXT((#7757,#7758,#7759))
REPRESENTATION_CONTEXT('','3D')
);
#7757=(
LENGTH_UNIT()
NAMED_UNIT(*)
SI_UNIT($,.METRE.)
);
#7758=(
NAMED_UNIT(*)
PLANE_ANGLE_UNIT()
SI_UNIT($,.RADIAN.)
);
#7759=(
NAMED_UNIT(*)
SI_UNIT($,.STERADIAN.)
SOLID_ANGLE_UNIT()
);
#7769=SHAPE_DEFINITION_REPRESENTATION(#7779,#7827);
#7779=PRODUCT_DEFINITION_SHAPE('',$,#7838);
#7827=SHAPE_REPRESENTATION('',(#5003),#7755);
#7828=PRODUCT_DEFINITION_CONTEXT('part definition',#7860,'design');
#7838=PRODUCT_DEFINITION('Corner Bottom Bracket',
'Corner Bottom Bracket',#7848,#7828);
#7848=PRODUCT_DEFINITION_FORMATION('',$,#7871);
#7860=APPLICATION_CONTEXT(
'Core Data for Automotive Mechanical Design Process');
#7861=PRODUCT_CONTEXT('part definition',#7860,'mechanical');
#7871=PRODUCT('Corner Bottom Bracket','Corner Bottom Bracket',
'LEGAL AND USAGE DISCLAIMER: this Data/Model is provided \X2\201C\X0\A
S IS\X2\201D\X0\ for informational and representational only. It is a 
geometric approximation and is NOT engineered, certified, or guarantee
d for dimensional accuracy, exact tolerances, or production-level prec
ision. Vendor disclaims all implied warranties including fitness for a
 particular purpose. DO NOT USE FOR DIRECT PHYSICAL MANUFACTURING, AUT
OMATED PRODUCTION, OR SAFETY-CRITICAL SYSTEMS without independent engi
neering verification and resolution of any design discrepancies.',(#7861));
#7878=PRESENTATION_STYLE_ASSIGNMENT((#7885));
#7885=SURFACE_STYLE_USAGE(.BOTH.,#7892);
#7892=SURFACE_SIDE_STYLE('',(#7899));
#7899=SURFACE_STYLE_FILL_AREA(#7906);
#7906=FILL_AREA_STYLE('Opaque(48,59,150)',(#7913));
#7913=FILL_AREA_STYLE_COLOUR('Opaque(48,59,150)',#7920);
#7920=COLOUR_RGB('Opaque(48,59,150)',0.188235294117647,0.231372549019608,
0.588235294117647);
ENDSEC;
END-ISO-10303-21;
